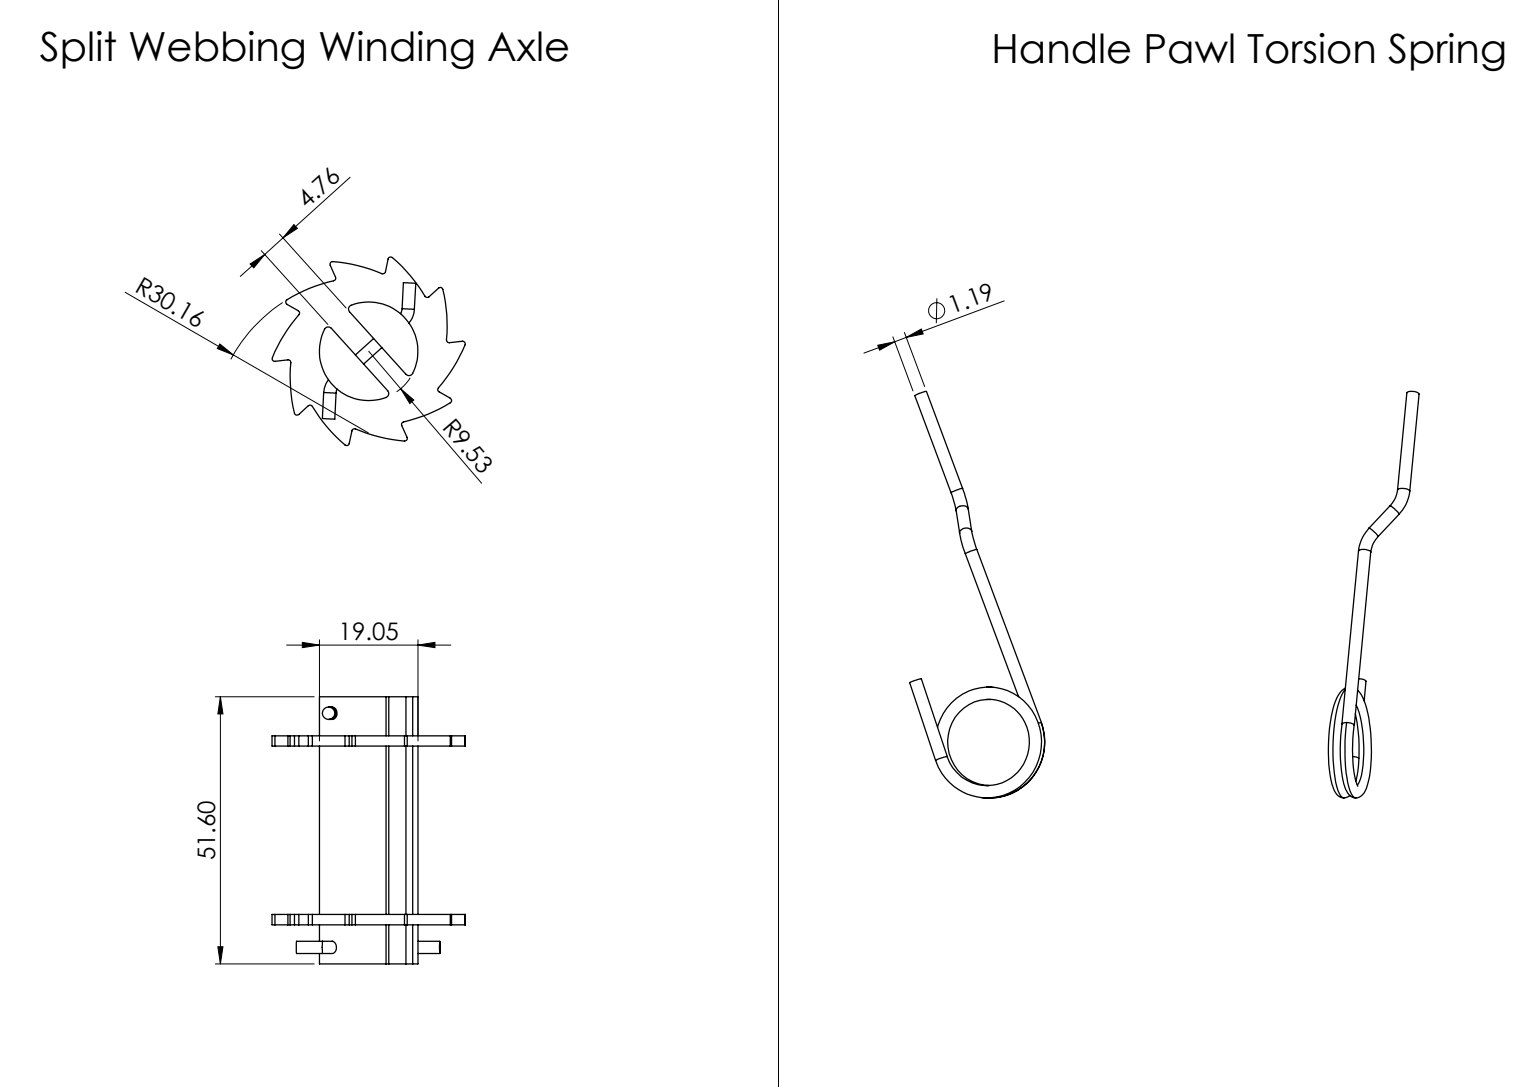
ISO-10303-21;
HEADER;
FILE_DESCRIPTION (('STEP AP214'),
    '1' );
FILE_NAME ('Split Webbing Winding Axle.step',
    '2026-10-09T14:10:49',
    ( '' ),
    ( '' ),
    'SwSTEP 2.0',
    'SolidWorks 2026',
    '' );
FILE_SCHEMA (( 'AUTOMOTIVE_DESIGN' ));
ENDSEC;

DATA;
#3=CIRCLE ( 'NONE', #8469, 0.5080000000000013394 ) ;
#24=CYLINDRICAL_SURFACE ( 'NONE', #13892, 30.16250000000000142 ) ;
#26=EDGE_CURVE ( 'NONE', #12400, #1617, #15318, .T. ) ;
#27=ORIENTED_EDGE ( 'NONE', *, *, #3397, .F. ) ;
#29=CARTESIAN_POINT ( 'NONE',  ( 53.08681243026497043, 37.69777154208443193, -16.72443647847455850 ) ) ;
#32=ORIENTED_EDGE ( 'NONE', *, *, #21036, .F. ) ;
#34=DIRECTION ( 'NONE',  ( 0.9943660382494290406, 0.000000000000000000, -0.1060008583745199739 ) ) ;
#36=EDGE_CURVE ( 'NONE', #1582, #17060, #15097, .T. ) ;
#41=ORIENTED_EDGE ( 'NONE', *, *, #3166, .F. ) ;
#52=EDGE_CURVE ( 'NONE', #9108, #5857, #17721, .T. ) ;
#53=CARTESIAN_POINT ( 'NONE',  ( 55.27198911326564001, 34.52875999999999834, 2.462719476673013830 ) ) ;
#55=ORIENTED_EDGE ( 'NONE', *, *, #21504, .F. ) ;
#56=ORIENTED_EDGE ( 'NONE', *, *, #17494, .T. ) ;
#58=CARTESIAN_POINT ( 'NONE',  ( 47.00675968526287818, 38.88803500000000213, -12.79836188810822328 ) ) ;
#62=ORIENTED_EDGE ( 'NONE', *, *, #7822, .T. ) ;
#64=VECTOR ( 'NONE', #8370, 1000.000000000000000 ) ;
#68=EDGE_CURVE ( 'NONE', #10096, #18019, #3909, .T. ) ;
#72=CYLINDRICAL_SURFACE ( 'NONE', #449, 30.16250000000000142 ) ;
#77=CYLINDRICAL_SURFACE ( 'NONE', #10849, 0.5080000000000005622 ) ;
#79=ORIENTED_EDGE ( 'NONE', *, *, #17597, .T. ) ;
#80=DIRECTION ( 'NONE',  ( 0.000000000000000000, 1.000000000000000000, 0.000000000000000000 ) ) ;
#89=ORIENTED_EDGE ( 'NONE', *, *, #190, .T. ) ;
#92=CARTESIAN_POINT ( 'NONE',  ( 39.27728671717661513, 34.52875999999999834, -23.95520057284206672 ) ) ;
#95=ORIENTED_EDGE ( 'NONE', *, *, #5447, .T. ) ;
#97=VERTEX_POINT ( 'NONE', #18926 ) ;
#101=DIRECTION ( 'NONE',  ( -0.6702301885068630005, 0.000000000000000000, -0.7421532822901580895 ) ) ;
#102=VECTOR ( 'NONE', #21181, 1000.000000000000114 ) ;
#106=FACE_OUTER_BOUND ( 'NONE', #16454, .T. ) ;
#107=VERTEX_POINT ( 'NONE', #482 ) ;
#110=CARTESIAN_POINT ( 'NONE',  ( 53.77834614425744064, -5.598900522968899729, -15.87027249378376936 ) ) ;
#112=CYLINDRICAL_SURFACE ( 'NONE', #2785, 0.5079999999999976756 ) ;
#114=EDGE_CURVE ( 'NONE', #97, #11029, #5668, .T. ) ;
#116=AXIS2_PLACEMENT_3D ( 'NONE', #2669, #1515, #18221 ) ;
#119=VERTEX_POINT ( 'NONE', #18820 ) ;
#137=EDGE_CURVE ( 'NONE', #6597, #20373, #21240, .T. ) ;
#139=DIRECTION ( 'NONE',  ( 0.05085730733808393328, 0.000000000000000000, -0.9987059298363656357 ) ) ;
#142=ORIENTED_EDGE ( 'NONE', *, *, #11602, .F. ) ;
#146=LINE ( 'NONE', #8543, #21177 ) ;
#147=VECTOR ( 'NONE', #5994, 1000.000000000000114 ) ;
#148=ORIENTED_EDGE ( 'NONE', *, *, #13327, .T. ) ;
#165=EDGE_CURVE ( 'NONE', #19859, #2625, #8173, .T. ) ;
#166=ORIENTED_EDGE ( 'NONE', *, *, #3462, .T. ) ;
#170=VECTOR ( 'NONE', #3329, 1000.000000000000000 ) ;
#173=LINE ( 'NONE', #16974, #9614 ) ;
#175=DIRECTION ( 'NONE',  ( -0.1060008583745224581, 0.000000000000000000, -0.9943660382494288186 ) ) ;
#180=VERTEX_POINT ( 'NONE', #9193 ) ;
#182=ADVANCED_FACE ( 'NONE', ( #3687 ), #8750, .T. ) ;
#185=LINE ( 'NONE', #17106, #9522 ) ;
#188=CYLINDRICAL_SURFACE ( 'NONE', #17566, 0.5080000000000007843 ) ;
#189=ORIENTED_EDGE ( 'NONE', *, *, #13845, .T. ) ;
#190=EDGE_CURVE ( 'NONE', #7494, #14487, #7555, .T. ) ;
#191=CARTESIAN_POINT ( 'NONE',  ( 53.25483508941461963, 42.06303499999999929, -5.879799058943532941 ) ) ;
#204=ORIENTED_EDGE ( 'NONE', *, *, #16141, .T. ) ;
#210=EDGE_CURVE ( 'NONE', #9895, #180, #14097, .T. ) ;
#213=DIRECTION ( 'NONE',  ( 0.2064631973582987667, 0.000000000000000000, -0.9784543669157944601 ) ) ;
#220=DIRECTION ( 'NONE',  ( 0.000000000000000000, -1.000000000000000000, 0.000000000000000000 ) ) ;
#221=CYLINDRICAL_SURFACE ( 'NONE', #1464, 0.5079999999999963434 ) ;
#225=CARTESIAN_POINT ( 'NONE',  ( 64.14292646034530776, 0.000000000000000000, -12.24881465648521939 ) ) ;
#229=CARTESIAN_POINT ( 'NONE',  ( 38.18512253410862201, -6.356984999999999886, -4.927479914652648674 ) ) ;
#248=CARTESIAN_POINT ( 'NONE',  ( 53.46798503507454825, 34.52875999999999834, 6.304111036318381878 ) ) ;
#250=FACE_OUTER_BOUND ( 'NONE', #17892, .T. ) ;
#251=ORIENTED_EDGE ( 'NONE', *, *, #17974, .F. ) ;
#253=AXIS2_PLACEMENT_3D ( 'NONE', #9461, #16230, #5826 ) ;
#261=EDGE_CURVE ( 'NONE', #11029, #831, #7657, .T. ) ;
#268=CIRCLE ( 'NONE', #3100, 1.190624999999997824 ) ;
#273=ORIENTED_EDGE ( 'NONE', *, *, #1147, .T. ) ;
#284=VECTOR ( 'NONE', #21016, 1000.000000000000000 ) ;
#286=EDGE_CURVE ( 'NONE', #20627, #1656, #19688, .T. ) ;
#293=CARTESIAN_POINT ( 'NONE',  ( 49.41195815393805901, -1.983739999999997838, -1.411525001868561224 ) ) ;
#297=ORIENTED_EDGE ( 'NONE', *, *, #14274, .F. ) ;
#299=DIRECTION ( 'NONE',  ( -0.5222415575336509797, 0.000000000000000000, -0.8527976052879290281 ) ) ;
#302=CARTESIAN_POINT ( 'NONE',  ( 32.18388890846549799, 32.54502000000000095, 1.507793899792891468 ) ) ;
#305=EDGE_LOOP ( 'NONE', ( #11333, #11552, #10599, #2404 ) ) ;
#312=ORIENTED_EDGE ( 'NONE', *, *, #165, .T. ) ;
#314=ORIENTED_EDGE ( 'NONE', *, *, #1169, .F. ) ;
#321=DIRECTION ( 'NONE',  ( 0.000000000000000000, 1.000000000000000000, 0.000000000000000000 ) ) ;
#325=CARTESIAN_POINT ( 'NONE',  ( 39.16413618835606769, 37.11476346399999926, -24.45043885672975392 ) ) ;
#330=DIRECTION ( 'NONE',  ( 0.000000000000000000, 1.000000000000000000, 0.000000000000000000 ) ) ;
#331=ORIENTED_EDGE ( 'NONE', *, *, #18672, .F. ) ;
#335=ORIENTED_EDGE ( 'NONE', *, *, #14252, .F. ) ;
#342=DIRECTION ( 'NONE',  ( -0.6496772031432439531, 0.000000000000000000, 0.7602101891687401691 ) ) ;
#343=AXIS2_PLACEMENT_3D ( 'NONE', #9406, #14736, #16073 ) ;
#346=VECTOR ( 'NONE', #19998, 1000.000000000000114 ) ;
#348=CARTESIAN_POINT ( 'NONE',  ( 38.84235393761607469, -5.162860800152350826, -4.075279525839791361 ) ) ;
#360=EDGE_CURVE ( 'NONE', #21347, #13814, #17389, .T. ) ;
#371=DIRECTION ( 'NONE',  ( -0.7421532822901579785, 0.000000000000000000, 0.6702301885068630005 ) ) ;
#373=CARTESIAN_POINT ( 'NONE',  ( 41.45112526417833010, -1.983739999999999837, 7.778260066349530710 ) ) ;
#392=DIRECTION ( 'NONE',  ( -0.7421532822901579785, 0.000000000000000000, 0.6702301885068628895 ) ) ;
#400=ORIENTED_EDGE ( 'NONE', *, *, #7902, .F. ) ;
#401=VECTOR ( 'NONE', #4265, 1000.000000000000000 ) ;
#404=ORIENTED_EDGE ( 'NONE', *, *, #18172, .T. ) ;
#405=LINE ( 'NONE', #7160, #11390 ) ;
#406=DIRECTION ( 'NONE',  ( -0.05085730733808142834, 0.000000000000000000, 0.9987059298363657467 ) ) ;
#409=CARTESIAN_POINT ( 'NONE',  ( 64.66604708500285881, 32.54502000000000095, -11.54913207920052720 ) ) ;
#412=ORIENTED_EDGE ( 'NONE', *, *, #11806, .F. ) ;
#424=LINE ( 'NONE', #13819, #15988 ) ;
#430=AXIS2_PLACEMENT_3D ( 'NONE', #13044, #6387, #21198 ) ;
#434=CIRCLE ( 'NONE', #1505, 0.5080000000000006732 ) ;
#439=DIRECTION ( 'NONE',  ( 0.8943161143440100380, 0.000000000000000000, 0.4474356798743612806 ) ) ;
#449=AXIS2_PLACEMENT_3D ( 'NONE', #12581, #16021, #15571 ) ;
#450=ORIENTED_EDGE ( 'NONE', *, *, #19358, .T. ) ;
#454=EDGE_CURVE ( 'NONE', #9720, #5388, #7845, .T. ) ;
#455=DIRECTION ( 'NONE',  ( 0.000000000000000000, 1.000000000000000000, 0.000000000000000000 ) ) ;
#459=CIRCLE ( 'NONE', #9260, 0.5079999999999973426 ) ;
#477=PLANE ( 'NONE',  #19448 ) ;
#482=CARTESIAN_POINT ( 'NONE',  ( 30.97944403357121956, -1.983739999999999837, -8.103300075789407586 ) ) ;
#485=ORIENTED_EDGE ( 'NONE', *, *, #3071, .F. ) ;
#493=CIRCLE ( 'NONE', #844, 1.190625000000000711 ) ;
#498=EDGE_CURVE ( 'NONE', #10812, #21347, #20182, .T. ) ;
#499=CARTESIAN_POINT ( 'NONE',  ( 53.14266576735298031, -7.546379553159687781, -16.66242751532464084 ) ) ;
#504=CARTESIAN_POINT ( 'NONE',  ( 52.39214030333819494, 39.62760010306434566, -17.41425762687993029 ) ) ;
#512=DIRECTION ( 'NONE',  ( 0.1060008583745224581, 0.000000000000000000, 0.9943660382494288186 ) ) ;
#521=AXIS2_PLACEMENT_3D ( 'NONE', #15161, #6738, #13502 ) ;
#523=DIRECTION ( 'NONE',  ( 0.7421532822901579785, 0.000000000000000000, -0.6702301885068630005 ) ) ;
#524=EDGE_LOOP ( 'NONE', ( #10286, #14452, #3255, #19034 ) ) ;
#525=CARTESIAN_POINT ( 'NONE',  ( 59.65121809612895731, 0.000000000000000000, -2.485718937265306572 ) ) ;
#527=CARTESIAN_POINT ( 'NONE',  ( 59.86950051480232560, -6.356984999999999886, -17.89453710146031185 ) ) ;
#530=ORIENTED_EDGE ( 'NONE', *, *, #8325, .F. ) ;
#531=ORIENTED_EDGE ( 'NONE', *, *, #4323, .T. ) ;
#535=VERTEX_POINT ( 'NONE', #17898 ) ;
#538=ORIENTED_EDGE ( 'NONE', *, *, #3166, .T. ) ;
#541=AXIS2_PLACEMENT_3D ( 'NONE', #1411, #17800, #2648 ) ;
#542=ORIENTED_EDGE ( 'NONE', *, *, #52, .F. ) ;
#546=CARTESIAN_POINT ( 'NONE',  ( 38.94885947252247860, -7.547248457916676756, -3.956611957470116625 ) ) ;
#551=DIRECTION ( 'NONE',  ( 0.000000000000000000, -1.000000000000000000, 0.000000000000000000 ) ) ;
#553=DIRECTION ( 'NONE',  ( -0.8583349619704310207, 0.000000000000000000, 0.5130897514657826175 ) ) ;
#557=ORIENTED_EDGE ( 'NONE', *, *, #19024, .T. ) ;
#563=ORIENTED_EDGE ( 'NONE', *, *, #17228, .T. ) ;
#568=CARTESIAN_POINT ( 'NONE',  ( 64.14292646034530776, -1.983739999999999837, -12.24881465648521939 ) ) ;
#570=EDGE_CURVE ( 'NONE', #16730, #6476, #8894, .T. ) ;
#575=ADVANCED_FACE ( 'NONE', ( #16250 ), #19549, .F. ) ;
#584=CARTESIAN_POINT ( 'NONE',  ( 52.91086381164393515, 2.586003464000000029, 3.812938856729753301 ) ) ;
#589=LINE ( 'NONE', #20695, #6002 ) ;
#597=EDGE_CURVE ( 'NONE', #14787, #535, #13511, .T. ) ;
#602=DIRECTION ( 'NONE',  ( 0.9129422336036122632, 0.000000000000000000, -0.4080888115384288528 ) ) ;
#609=ORIENTED_EDGE ( 'NONE', *, *, #4647, .F. ) ;
#611=CARTESIAN_POINT ( 'NONE',  ( 30.25543876212147509, 34.52875999999999834, -19.39939755251907272 ) ) ;
#614=FACE_OUTER_BOUND ( 'NONE', #18678, .T. ) ;
#619=CYLINDRICAL_SURFACE ( 'NONE', #19701, 30.16249999999999076 ) ;
#620=EDGE_CURVE ( 'NONE', #8192, #8377, #16467, .T. ) ;
#621=EDGE_LOOP ( 'NONE', ( #5754, #17722, #15374, #17996, #9493, #4829, #6803, #12935, #19285, #5126, #563, #5731, #12820, #9699, #14120, #19790, #20475, #19543, #9154, #13893, #19426, #8672, #3701, #4027, #204, #17065, #19652, #9741, #16692, #2515, #19472, #8946, #13944, #4403, #14015, #10589, #1724, #609, #18551, #13398 ) ) ;
#625=CARTESIAN_POINT ( 'NONE',  ( 59.80894853325292360, -6.356984999999999886, -16.70545285374888778 ) ) ;
#633=AXIS2_PLACEMENT_3D ( 'NONE', #13523, #13632, #8307 ) ;
#651=ORIENTED_EDGE ( 'NONE', *, *, #18149, .F. ) ;
#661=DIRECTION ( 'NONE',  ( 0.07875956036501312318, 0.000000000000000000, -0.9968936410927243807 ) ) ;
#667=CIRCLE ( 'NONE', #3491, 1.984375000000000000 ) ;
#672=CARTESIAN_POINT ( 'NONE',  ( 37.13209340688868565, -6.356984999999999886, -3.529402718062123689 ) ) ;
#673=VECTOR ( 'NONE', #3578, 1000.000000000000000 ) ;
#683=DIRECTION ( 'NONE',  ( 0.000000000000000000, 1.000000000000000000, 0.000000000000000000 ) ) ;
#684=CARTESIAN_POINT ( 'NONE',  ( 38.23013820809905638, -9.531985000000000596, -14.22485453658974031 ) ) ;
#687=AXIS2_PLACEMENT_3D ( 'NONE', #15125, #6696, #20168 ) ;
#689=ORIENTED_EDGE ( 'NONE', *, *, #13845, .F. ) ;
#690=DIRECTION ( 'NONE',  ( -0.000000000000000000, -1.000000000000000000, 0.000000000000000000 ) ) ;
#704=DIRECTION ( 'NONE',  ( 0.9784543669157820256, 0.000000000000000000, 0.2064631973583577473 ) ) ;
#709=VECTOR ( 'NONE', #2797, 1000.000000000000000 ) ;
#713=FACE_OUTER_BOUND ( 'NONE', #15999, .T. ) ;
#715=ADVANCED_FACE ( 'NONE', ( #13584 ), #1729, .F. ) ;
#718=ADVANCED_FACE ( 'NONE', ( #1946 ), #18430, .T. ) ;
#719=ADVANCED_FACE ( 'NONE', ( #3305 ), #10243, .F. ) ;
#723=VERTEX_POINT ( 'NONE', #3504 ) ;
#734=DIRECTION ( 'NONE',  ( 0.3928209820863007851, 0.000000000000000000, -0.9196149607486571176 ) ) ;
#741=ORIENTED_EDGE ( 'NONE', *, *, #1772, .T. ) ;
#745=LINE ( 'NONE', #16241, #21205 ) ;
#746=CIRCLE ( 'NONE', #9211, 0.5079999999999996740 ) ;
#747=EDGE_LOOP ( 'NONE', ( #450, #19069, #6393, #18964 ) ) ;
#753=ORIENTED_EDGE ( 'NONE', *, *, #1834, .F. ) ;
#756=CIRCLE ( 'NONE', #19475, 0.5079999999999985638 ) ;
#758=EDGE_CURVE ( 'NONE', #20373, #1329, #18433, .T. ) ;
#763=AXIS2_PLACEMENT_3D ( 'NONE', #1873, #5290, #4872 ) ;
#770=CARTESIAN_POINT ( 'NONE',  ( 55.33978576324753362, 0.000000000000000000, -23.05096232720518756 ) ) ;
#774=DIRECTION ( 'NONE',  ( 0.000000000000000000, 1.000000000000000000, 0.000000000000000000 ) ) ;
#780=DIRECTION ( 'NONE',  ( 0.000000000000000000, 1.000000000000000000, 0.000000000000000000 ) ) ;
#781=AXIS2_PLACEMENT_3D ( 'NONE', #4089, #977, #12506 ) ;
#782=AXIS2_PLACEMENT_3D ( 'NONE', #19094, #1965, #3522 ) ;
#784=DIRECTION ( 'NONE',  ( 0.000000000000000000, 1.000000000000000000, 0.000000000000000000 ) ) ;
#789=AXIS2_PLACEMENT_3D ( 'NONE', #10505, #19118, #10616 ) ;
#790=CARTESIAN_POINT ( 'NONE',  ( 38.23013820809905638, 42.06303499999999929, -14.22485453658974031 ) ) ;
#791=DIRECTION ( 'NONE',  ( -0.4080888115384288528, 0.000000000000000000, -0.9129422336036122632 ) ) ;
#804=DIRECTION ( 'NONE',  ( 0.000000000000000000, 1.000000000000000000, 0.000000000000000000 ) ) ;
#806=VECTOR ( 'NONE', #16119, 1000.000000000000000 ) ;
#809=DIRECTION ( 'NONE',  ( 0.000000000000000000, 1.000000000000000000, 0.000000000000000000 ) ) ;
#819=ORIENTED_EDGE ( 'NONE', *, *, #16382, .T. ) ;
#824=DIRECTION ( 'NONE',  ( -0.1060008583745224581, 0.000000000000000000, -0.9943660382494288186 ) ) ;
#826=PRODUCT_DEFINITION_CONTEXT ( 'detailed design', #18349, 'design' ) ;
#830=CARTESIAN_POINT ( 'NONE',  ( 52.22368883687065022, 39.20681492737163154, -17.56171959381228476 ) ) ;
#831=VERTEX_POINT ( 'NONE', #12016 ) ;
#834=CIRCLE ( 'NONE', #8244, 30.16249999999998721 ) ;
#837=CARTESIAN_POINT ( 'NONE',  ( 59.52193197173441774, -1.983739999999999837, -3.260183413611184911 ) ) ;
#838=ORIENTED_EDGE ( 'NONE', *, *, #9399, .T. ) ;
#841=ORIENTED_EDGE ( 'NONE', *, *, #10075, .F. ) ;
#844=AXIS2_PLACEMENT_3D ( 'NONE', #8969, #14195, #20909 ) ;
#850=ADVANCED_FACE ( 'NONE', ( #10135 ), #72, .T. ) ;
#855=LINE ( 'NONE', #17779, #102 ) ;
#856=CARTESIAN_POINT ( 'NONE',  ( 38.94885947252247860, -7.547248457916676756, -3.956611957470116625 ) ) ;
#858=ORIENTED_EDGE ( 'NONE', *, *, #4636, .F. ) ;
#859=ORIENTED_EDGE ( 'NONE', *, *, #3535, .T. ) ;
#863=ORIENTED_EDGE ( 'NONE', *, *, #16462, .T. ) ;
#866=ORIENTED_EDGE ( 'NONE', *, *, #19505, .T. ) ;
#867=VECTOR ( 'NONE', #15872, 1000.000000000000000 ) ;
#872=EDGE_CURVE ( 'NONE', #8553, #5503, #6086, .T. ) ;
#874=CARTESIAN_POINT ( 'NONE',  ( 59.55063415577301811, 32.54502000000000095, -22.52230776719629191 ) ) ;
#877=VERTEX_POINT ( 'NONE', #9239 ) ;
#881=CYLINDRICAL_SURFACE ( 'NONE', #9261, 1.190624999999997824 ) ;
#890=VECTOR ( 'NONE', #9483, 1000.000000000000000 ) ;
#895=CARTESIAN_POINT ( 'NONE',  ( 59.90456643211351917, 37.11476346399999926, -2.926035437812116946 ) ) ;
#900=DIRECTION ( 'NONE',  ( 0.000000000000000000, 1.000000000000000000, 0.000000000000000000 ) ) ;
#906=FACE_OUTER_BOUND ( 'NONE', #1227, .T. ) ;
#909=DIRECTION ( 'NONE',  ( 0.000000000000000000, -1.000000000000000000, -0.000000000000000000 ) ) ;
#914=EDGE_LOOP ( 'NONE', ( #6101, #19962 ) ) ;
#917=LINE ( 'NONE', #20928, #8769 ) ;
#923=CARTESIAN_POINT ( 'NONE',  ( 53.00421038040393995, 0.000000000000000000, 6.511420152579801446 ) ) ;
#924=ORIENTED_EDGE ( 'NONE', *, *, #3296, .T. ) ;
#929=CARTESIAN_POINT ( 'NONE',  ( 53.50176854207381183, -7.446663216667899654, -16.23620094008295567 ) ) ;
#930=CARTESIAN_POINT ( 'NONE',  ( 39.90410341501912939, 39.21273375806297423, -3.030981210009983329 ) ) ;
#933=ORIENTED_EDGE ( 'NONE', *, *, #3535, .F. ) ;
#934=CARTESIAN_POINT ( 'NONE',  ( 52.55824432597118800, 39.85392714130129832, -17.26273071540813930 ) ) ;
#935=ORIENTED_EDGE ( 'NONE', *, *, #8739, .T. ) ;
#940=CARTESIAN_POINT ( 'NONE',  ( 38.23013820809905638, 109.3223030719999969, -14.22485453658974031 ) ) ;
#948=ORIENTED_EDGE ( 'NONE', *, *, #19907, .F. ) ;
#953=CYLINDRICAL_SURFACE ( 'NONE', #8579, 1.190624999999999822 ) ;
#954=DIRECTION ( 'NONE',  ( 0.000000000000000000, 1.000000000000000000, 0.000000000000000000 ) ) ;
#964=EDGE_CURVE ( 'NONE', #12607, #1384, #20908, .T. ) ;
#965=CIRCLE ( 'NONE', #18263, 4.365624999999999645 ) ;
#968=VERTEX_POINT ( 'NONE', #12242 ) ;
#970=FACE_OUTER_BOUND ( 'NONE', #7558, .T. ) ;
#976=DIRECTION ( 'NONE',  ( -0.9987059298363656357, 0.000000000000000000, -0.05085730733808393328 ) ) ;
#977=DIRECTION ( 'NONE',  ( 0.000000000000000000, 1.000000000000000000, 0.000000000000000000 ) ) ;
#981=ORIENTED_EDGE ( 'NONE', *, *, #3143, .F. ) ;
#991=DIRECTION ( 'NONE',  ( 0.000000000000000000, 1.000000000000000000, 0.000000000000000000 ) ) ;
#994=VECTOR ( 'NONE', #12853, 1000.000000000000000 ) ;
#1006=LINE ( 'NONE', #14849, #1063 ) ;
#1009=EDGE_CURVE ( 'NONE', #968, #19531, #14254, .T. ) ;
#1011=CARTESIAN_POINT ( 'NONE',  ( 61.65536943582333151, 0.000000000000000000, -11.98363747855214712 ) ) ;
#1021=VERTEX_POINT ( 'NONE', #8792 ) ;
#1028=DIRECTION ( 'NONE',  ( 0.000000000000000000, -1.000000000000000000, -0.000000000000000000 ) ) ;
#1030=DIRECTION ( 'NONE',  ( 0.000000000000000000, -1.000000000000000000, -0.000000000000000000 ) ) ;
#1033=EDGE_CURVE ( 'NONE', #1535, #12957, #405, .T. ) ;
#1034=VECTOR ( 'NONE', #2801, 1000.000000000000114 ) ;
#1038=DIRECTION ( 'NONE',  ( 0.000000000000000000, -1.000000000000000000, -0.000000000000000000 ) ) ;
#1039=DIRECTION ( 'NONE',  ( 0.000000000000000000, 1.000000000000000000, 0.000000000000000000 ) ) ;
#1042=CARTESIAN_POINT ( 'NONE',  ( 53.10651001381376091, 37.69740999999999786, -16.70269254552787075 ) ) ;
#1046=LINE ( 'NONE', #9338, #10598 ) ;
#1050=VERTEX_POINT ( 'NONE', #12996 ) ;
#1060=EDGE_CURVE ( 'NONE', #11223, #2583, #1466, .T. ) ;
#1063=VECTOR ( 'NONE', #5977, 1000.000000000000114 ) ;
#1065=VECTOR ( 'NONE', #13779, 1000.000000000000000 ) ;
#1068=VERTEX_POINT ( 'NONE', #18065 ) ;
#1074=VERTEX_POINT ( 'NONE', #6656 ) ;
#1075=AXIS2_PLACEMENT_3D ( 'NONE', #5417, #7209, #5200 ) ;
#1078=AXIS2_PLACEMENT_3D ( 'NONE', #1933, #7356, #5576 ) ;
#1081=CARTESIAN_POINT ( 'NONE',  ( 39.54651519818619221, 37.91656218874415885, -3.347550931093328686 ) ) ;
#1089=TOROIDAL_SURFACE ( 'NONE', #15240, 3.174999999999999822, 1.190625000000000044 ) ;
#1095=ORIENTED_EDGE ( 'NONE', *, *, #21176, .F. ) ;
#1099=CARTESIAN_POINT ( 'NONE',  ( 36.80301088673436283, 0.000000000000000000, -23.10021947667301134 ) ) ;
#1112=DIRECTION ( 'NONE',  ( -0.9129422336036127072, 0.000000000000000000, 0.4080888115384278536 ) ) ;
#1116=EDGE_CURVE ( 'NONE', #20800, #15003, #18486, .T. ) ;
#1117=VERTEX_POINT ( 'NONE', #11433 ) ;
#1123=DIRECTION ( 'NONE',  ( -0.3928209820863007296, 0.000000000000000000, 0.9196149607486571176 ) ) ;
#1124=AXIS2_PLACEMENT_3D ( 'NONE', #1554, #6631, #4975 ) ;
#1126=VERTEX_POINT ( 'NONE', #8214 ) ;
#1128=AXIS2_PLACEMENT_3D ( 'NONE', #3087, #5065, #9811 ) ;
#1136=CARTESIAN_POINT ( 'NONE',  ( 39.88301061098722755, 0.000000000000000000, -24.08706006053352411 ) ) ;
#1137=EDGE_CURVE ( 'NONE', #8133, #7171, #5738, .T. ) ;
#1144=CARTESIAN_POINT ( 'NONE',  ( 45.99559936598748777, 34.52875999999999834, 5.449572532947073000 ) ) ;
#1146=AXIS2_PLACEMENT_3D ( 'NONE', #16018, #14139, #3837 ) ;
#1147=EDGE_CURVE ( 'NONE', #1819, #7588, #4799, .T. ) ;
#1163=CARTESIAN_POINT ( 'NONE',  ( 49.79678389823170903, 34.52875999999999834, -28.13445659451038594 ) ) ;
#1166=ADVANCED_FACE ( 'NONE', ( #13103 ), #1350, .T. ) ;
#1169=EDGE_CURVE ( 'NONE', #1190, #8553, #3129, .T. ) ;
#1174=AXIS2_PLACEMENT_3D ( 'NONE', #20913, #5776, #4011 ) ;
#1175=CARTESIAN_POINT ( 'NONE',  ( 38.76261520251843251, 37.72836252664282597, -4.168749548257426163 ) ) ;
#1181=CARTESIAN_POINT ( 'NONE',  ( 38.82016491058538321, 42.06303499999999929, -14.75770094105646812 ) ) ;
#1183=ORIENTED_EDGE ( 'NONE', *, *, #18457, .T. ) ;
#1184=DIRECTION ( 'NONE',  ( 0.000000000000000000, -1.000000000000000000, -0.000000000000000000 ) ) ;
#1190=VERTEX_POINT ( 'NONE', #3244 ) ;
#1193=ADVANCED_FACE ( 'NONE', ( #6330 ), #3031, .F. ) ;
#1197=CIRCLE ( 'NONE', #13575, 0.7950199999999993938 ) ;
#1198=CARTESIAN_POINT ( 'NONE',  ( 38.18512253410862201, -6.356984999999999886, -4.927479914652648674 ) ) ;
#1199=CYLINDRICAL_SURFACE ( 'NONE', #4030, 1.190625000000000488 ) ;
#1206=DIRECTION ( 'NONE',  ( -0.3542738219355860418, 0.000000000000000000, -0.9351417320872557060 ) ) ;
#1207=CARTESIAN_POINT ( 'NONE',  ( 53.84912356528904809, 38.73144433068016923, -15.76890250127162219 ) ) ;
#1209=VERTEX_POINT ( 'NONE', #4689 ) ;
#1217=CARTESIAN_POINT ( 'NONE',  ( 32.96560389001691505, 0.000000000000000000, -17.84002872454335886 ) ) ;
#1223=CARTESIAN_POINT ( 'NONE',  ( 61.65536943582333151, -1.983739999999999837, -11.98363747855214712 ) ) ;
#1226=DIRECTION ( 'NONE',  ( -0.4987171968201974948, 0.000000000000000000, 0.8667647648559581031 ) ) ;
#1227=EDGE_LOOP ( 'NONE', ( #9061, #2863, #19485, #6400 ) ) ;
#1229=DIRECTION ( 'NONE',  ( 0.000000000000000000, 1.000000000000000000, 0.000000000000000000 ) ) ;
#1232=CIRCLE ( 'NONE', #9341, 30.16249999999999076 ) ;
#1233=CARTESIAN_POINT ( 'NONE',  ( 36.80301088673436283, 32.54502000000000095, -23.10021947667301134 ) ) ;
#1234=ORIENTED_EDGE ( 'NONE', *, *, #7163, .T. ) ;
#1235=DIRECTION ( 'NONE',  ( -0.2227372614607789347, 0.000000000000000000, -0.9748785115884710528 ) ) ;
#1241=DIRECTION ( 'NONE',  ( 0.4987171968201974948, 0.000000000000000000, -0.8667647648559581031 ) ) ;
#1244=EDGE_CURVE ( 'NONE', #3969, #9951, #4333, .T. ) ;
#1245=ADVANCED_FACE ( 'NONE', ( #4575 ), #11315, .T. ) ;
#1247=DIRECTION ( 'NONE',  ( 0.7532174416907910786, 0.000000000000000000, 0.6577716059034319773 ) ) ;
#1251=CARTESIAN_POINT ( 'NONE',  ( 35.15748561355322011, -1.983739999999999837, 0.3244898641346534163 ) ) ;
#1254=CARTESIAN_POINT ( 'NONE',  ( 39.22869158989735894, 40.05999463121278836, -3.656238088543281695 ) ) ;
#1258=EDGE_CURVE ( 'NONE', #8259, #8918, #16003, .T. ) ;
#1263=DIRECTION ( 'NONE',  ( -0.6702301885068630005, 0.000000000000000000, -0.7421532822901579785 ) ) ;
#1265=PLANE ( 'NONE',  #7770 ) ;
#1271=EDGE_CURVE ( 'NONE', #1509, #15569, #7226, .T. ) ;
#1277=ADVANCED_FACE ( 'NONE', ( #20683 ), #18810, .T. ) ;
#1278=CARTESIAN_POINT ( 'NONE',  ( 38.22590828043067290, 38.73299043104906758, -4.868551855887884194 ) ) ;
#1283=ORIENTED_EDGE ( 'NONE', *, *, #9674, .T. ) ;
#1284=FACE_OUTER_BOUND ( 'NONE', #12717, .T. ) ;
#1287=ORIENTED_EDGE ( 'NONE', *, *, #8664, .T. ) ;
#1288=EDGE_CURVE ( 'NONE', #2524, #17693, #18696, .T. ) ;
#1289=ORIENTED_EDGE ( 'NONE', *, *, #16141, .F. ) ;
#1293=ORIENTED_EDGE ( 'NONE', *, *, #4679, .T. ) ;
#1296=ORIENTED_EDGE ( 'NONE', *, *, #11249, .T. ) ;
#1301=PLANE ( 'NONE',  #11805 ) ;
#1304=ORIENTED_EDGE ( 'NONE', *, *, #18290, .T. ) ;
#1306=CARTESIAN_POINT ( 'NONE',  ( 46.03750000000000142, 0.000000000000000000, -10.31874999999999964 ) ) ;
#1312=ORIENTED_EDGE ( 'NONE', *, *, #21259, .T. ) ;
#1315=CARTESIAN_POINT ( 'NONE',  ( 64.19677489640052670, 32.54502000000000095, -11.74367670905533423 ) ) ;
#1323=AXIS2_PLACEMENT_3D ( 'NONE', #10611, #20419, #3763 ) ;
#1325=DIRECTION ( 'NONE',  ( 0.000000000000000000, -1.000000000000000000, -0.000000000000000000 ) ) ;
#1329=VERTEX_POINT ( 'NONE', #6092 ) ;
#1332=FACE_OUTER_BOUND ( 'NONE', #2278, .T. ) ;
#1340=AXIS2_PLACEMENT_3D ( 'NONE', #2556, #12406, #17593 ) ;
#1342=CARTESIAN_POINT ( 'NONE',  ( 53.25483508941461963, -9.531985000000000596, -5.879799058943532941 ) ) ;
#1350=CYLINDRICAL_SURFACE ( 'NONE', #3619, 0.5079999999999965654 ) ;
#1353=LINE ( 'NONE', #21593, #9596 ) ;
#1357=CARTESIAN_POINT ( 'NONE',  ( 61.60152099976809126, -1.983739999999999837, -12.48877542598203405 ) ) ;
#1358=CARTESIAN_POINT ( 'NONE',  ( 64.66604708500285881, -1.983739999999999837, -11.54913207920052720 ) ) ;
#1362=CARTESIAN_POINT ( 'NONE',  ( 61.56621290189396944, 34.52875999999999834, -0.7977859469341201937 ) ) ;
#1363=CARTESIAN_POINT ( 'NONE',  ( 52.55890053324426248, 37.92160077886185121, -17.26210851293683390 ) ) ;
#1370=CARTESIAN_POINT ( 'NONE',  ( 42.79471501377724252, 34.52875999999999834, 5.049205022181460834 ) ) ;
#1382=( NAMED_UNIT ( * ) PLANE_ANGLE_UNIT ( ) SI_UNIT ( $, .RADIAN. ) );
#1383=ADVANCED_FACE ( 'NONE', ( #906 ), #2456, .F. ) ;
#1384=VERTEX_POINT ( 'NONE', #2567 ) ;
#1398=ORIENTED_EDGE ( 'NONE', *, *, #18691, .F. ) ;
#1400=CIRCLE ( 'NONE', #10270, 0.5080000000000016724 ) ;
#1411=CARTESIAN_POINT ( 'NONE',  ( 46.07940063401251507, 0.000000000000000000, -26.08707253294707229 ) ) ;
#1415=EDGE_CURVE ( 'NONE', #7335, #3338, #5734, .T. ) ;
#1416=LINE ( 'NONE', #8050, #20933 ) ;
#1419=CARTESIAN_POINT ( 'NONE',  ( 53.57639120092643736, 39.84016936695267930, -16.14136963297940497 ) ) ;
#1425=VERTEX_POINT ( 'NONE', #19582 ) ;
#1430=EDGE_CURVE ( 'NONE', #12951, #877, #19467, .T. ) ;
#1435=DIRECTION ( 'NONE',  ( -0.7421532822901579785, 0.000000000000000000, 0.6702301885068630005 ) ) ;
#1456=DIRECTION ( 'NONE',  ( 0.7421532822901579785, 0.000000000000000000, -0.6702301885068630005 ) ) ;
#1459=AXIS2_PLACEMENT_3D ( 'NONE', #6311, #9520, #1123 ) ;
#1463=CARTESIAN_POINT ( 'NONE',  ( 52.79771328282338771, 0.000000000000000000, 3.317700572842066986 ) ) ;
#1464=AXIS2_PLACEMENT_3D ( 'NONE', #18570, #6861, #6961 ) ;
#1465=AXIS2_PLACEMENT_3D ( 'NONE', #8510, #8080, #8195 ) ;
#1466=LINE ( 'NONE', #6450, #2210 ) ;
#1467=LINE ( 'NONE', #7779, #17824 ) ;
#1470=CARTESIAN_POINT ( 'NONE',  ( 54.55586098912687731, 42.06303499999999929, -6.056925149195119040 ) ) ;
#1471=AXIS2_PLACEMENT_3D ( 'NONE', #4974, #20002, #14962 ) ;
#1475=LINE ( 'NONE', #8221, #9766 ) ;
#1482=CYLINDRICAL_SURFACE ( 'NONE', #18394, 0.7950199999999985057 ) ;
#1485=ORIENTED_EDGE ( 'NONE', *, *, #2953, .T. ) ;
#1488=CIRCLE ( 'NONE', #9595, 30.16249999999999076 ) ;
#1505=AXIS2_PLACEMENT_3D ( 'NONE', #9439, #21375, #6231 ) ;
#1508=CARTESIAN_POINT ( 'NONE',  ( 52.65345379380355695, 37.69740999999999786, -16.29354262597941982 ) ) ;
#1509=VERTEX_POINT ( 'NONE', #21425 ) ;
#1511=ORIENTED_EDGE ( 'NONE', *, *, #4111, .T. ) ;
#1512=VERTEX_POINT ( 'NONE', #13051 ) ;
#1513=AXIS2_PLACEMENT_3D ( 'NONE', #12024, #14937, #10368 ) ;
#1514=EDGE_CURVE ( 'NONE', #18977, #107, #1416, .T. ) ;
#1515=DIRECTION ( 'NONE',  ( 0.000000000000000000, 1.000000000000000000, 0.000000000000000000 ) ) ;
#1516=EDGE_LOOP ( 'NONE', ( #5996, #3693 ) ) ;
#1527=DIRECTION ( 'NONE',  ( 0.8667647648559581031, 0.000000000000000000, 0.4987171968201974948 ) ) ;
#1529=CARTESIAN_POINT ( 'NONE',  ( 53.57721252000833800, 37.93694508125481235, -16.14030231556136741 ) ) ;
#1531=ORIENTED_EDGE ( 'NONE', *, *, #360, .T. ) ;
#1535=VERTEX_POINT ( 'NONE', #11049 ) ;
#1536=ADVANCED_FACE ( 'NONE', ( #12712 ), #21206, .F. ) ;
#1538=ORIENTED_EDGE ( 'NONE', *, *, #8761, .F. ) ;
#1544=AXIS2_PLACEMENT_3D ( 'NONE', #5510, #321, #15717 ) ;
#1546=DIRECTION ( 'NONE',  ( -0.6702301885068638887, 0.000000000000000000, -0.7421532822901570903 ) ) ;
#1549=DIRECTION ( 'NONE',  ( 0.9129422336036127072, 0.000000000000000000, -0.4080888115384278536 ) ) ;
#1554=CARTESIAN_POINT ( 'NONE',  ( 47.80475250345301674, -6.356984999999999886, -11.91473563638243327 ) ) ;
#1556=ORIENTED_EDGE ( 'NONE', *, *, #5973, .T. ) ;
#1562=AXIS2_PLACEMENT_3D ( 'NONE', #2373, #4142, #10880 ) ;
#1566=FACE_OUTER_BOUND ( 'NONE', #20603, .T. ) ;
#1567=CARTESIAN_POINT ( 'NONE',  ( 41.78116128337411794, 34.52875999999999834, 7.392073290253172502 ) ) ;
#1571=ORIENTED_EDGE ( 'NONE', *, *, #1634, .T. ) ;
#1574=AXIS2_PLACEMENT_3D ( 'NONE', #19977, #2980, #16575 ) ;
#1577=CARTESIAN_POINT ( 'NONE',  ( 41.71184157647478230, 38.88803500000000213, -2.134205101306931862 ) ) ;
#1582=VERTEX_POINT ( 'NONE', #19437 ) ;
#1598=ORIENTED_EDGE ( 'NONE', *, *, #13900, .F. ) ;
#1603=AXIS2_PLACEMENT_3D ( 'NONE', #8646, #3680, #10425 ) ;
#1605=CYLINDRICAL_SURFACE ( 'NONE', #14505, 30.16250000000000497 ) ;
#1606=ORIENTED_EDGE ( 'NONE', *, *, #68, .T. ) ;
#1610=CARTESIAN_POINT ( 'NONE',  ( 53.95242430215955665, 38.88803500000000213, -23.51676380836238067 ) ) ;
#1611=ORIENTED_EDGE ( 'NONE', *, *, #18172, .F. ) ;
#1613=ADVANCED_FACE ( 'NONE', ( #17904 ), #3086, .F. ) ;
#1617=VERTEX_POINT ( 'NONE', #7833 ) ;
#1620=ORIENTED_EDGE ( 'NONE', *, *, #12085, .F. ) ;
#1621=CARTESIAN_POINT ( 'NONE',  ( 38.23013820809905638, 34.52875999999999834, -14.22485453658974031 ) ) ;
#1623=CARTESIAN_POINT ( 'NONE',  ( 49.72033008250774344, 42.06303499999999929, -2.687827786179598277 ) ) ;
#1627=DIRECTION ( 'NONE',  ( 0.5222415575336524229, 0.000000000000000000, 0.8527976052879281399 ) ) ;
#1634=EDGE_CURVE ( 'NONE', #1329, #15472, #9617, .T. ) ;
#1636=DIRECTION ( 'NONE',  ( 0.000000000000000000, 1.000000000000000000, 0.000000000000000000 ) ) ;
#1640=AXIS2_PLACEMENT_3D ( 'NONE', #18596, #3466, #10200 ) ;
#1650=EDGE_LOOP ( 'NONE', ( #3417, #10618, #16697, #7905 ) ) ;
#1653=CARTESIAN_POINT ( 'NONE',  ( 52.89438837027574181, -7.516544198863053694, -16.93158128026265885 ) ) ;
#1656=VERTEX_POINT ( 'NONE', #191 ) ;
#1670=EDGE_CURVE ( 'NONE', #1656, #13806, #15669, .T. ) ;
#1675=DIRECTION ( 'NONE',  ( 0.000000000000000000, 1.000000000000000000, 0.000000000000000000 ) ) ;
#1679=VECTOR ( 'NONE', #5420, 1000.000000000000000 ) ;
#1680=ORIENTED_EDGE ( 'NONE', *, *, #21692, .T. ) ;
#1681=EDGE_CURVE ( 'NONE', #14418, #11144, #11913, .T. ) ;
#1690=ORIENTED_EDGE ( 'NONE', *, *, #5153, .F. ) ;
#1698=VERTEX_POINT ( 'NONE', #16886 ) ;
#1701=EDGE_CURVE ( 'NONE', #13851, #8918, #7179, .T. ) ;
#1716=AXIS2_PLACEMENT_3D ( 'NONE', #4854, #11488, #15146 ) ;
#1724=ORIENTED_EDGE ( 'NONE', *, *, #15650, .T. ) ;
#1725=DIRECTION ( 'NONE',  ( 0.9959941601142464629, 0.000000000000000000, 0.08941830359784661009 ) ) ;
#1726=ORIENTED_EDGE ( 'NONE', *, *, #19630, .T. ) ;
#1727=EDGE_CURVE ( 'NONE', #6920, #17175, #14614, .T. ) ;
#1729=CYLINDRICAL_SURFACE ( 'NONE', #21257, 0.5080000000000014504 ) ;
#1732=FACE_OUTER_BOUND ( 'NONE', #14774, .T. ) ;
#1735=VERTEX_POINT ( 'NONE', #20293 ) ;
#1742=ORIENTED_EDGE ( 'NONE', *, *, #19248, .F. ) ;
#1746=ORIENTED_EDGE ( 'NONE', *, *, #14225, .F. ) ;
#1760=DIRECTION ( 'NONE',  ( 0.9784543669157820256, 0.000000000000000000, 0.2064631973583577473 ) ) ;
#1764=VECTOR ( 'NONE', #9628, 1000.000000000000000 ) ;
#1767=CIRCLE ( 'NONE', #6716, 0.5080000000000000071 ) ;
#1772=EDGE_CURVE ( 'NONE', #4527, #1656, #18757, .T. ) ;
#1773=CARTESIAN_POINT ( 'NONE',  ( 39.58386072796550081, 38.88803500000000213, -4.490541772578183100 ) ) ;
#1777=EDGE_CURVE ( 'NONE', #13169, #13930, #7878, .T. ) ;
#1787=FACE_OUTER_BOUND ( 'NONE', #13799, .T. ) ;
#1790=VECTOR ( 'NONE', #4709, 1000.000000000000000 ) ;
#1795=LINE ( 'NONE', #17058, #10488 ) ;
#1803=EDGE_CURVE ( 'NONE', #16972, #11670, #19980, .T. ) ;
#1806=VECTOR ( 'NONE', #9637, 1000.000000000000000 ) ;
#1807=CIRCLE ( 'NONE', #18754, 0.5079999999999985638 ) ;
#1808=AXIS2_PLACEMENT_3D ( 'NONE', #10508, #6965, #15505 ) ;
#1811=EDGE_CURVE ( 'NONE', #7476, #17693, #13183, .T. ) ;
#1816=EDGE_CURVE ( 'NONE', #6920, #19435, #12114, .T. ) ;
#1819=VERTEX_POINT ( 'NONE', #20194 ) ;
#1822=AXIS2_PLACEMENT_3D ( 'NONE', #12937, #19751, #16572 ) ;
#1823=ORIENTED_EDGE ( 'NONE', *, *, #16213, .F. ) ;
#1828=CARTESIAN_POINT ( 'NONE',  ( 38.96848998618624904, -7.547609999999999708, -3.934807454472129429 ) ) ;
#1833=EDGE_CURVE ( 'NONE', #8981, #14185, #11815, .T. ) ;
#1834=EDGE_CURVE ( 'NONE', #7504, #3737, #15369, .T. ) ;
#1842=VECTOR ( 'NONE', #10307, 1000.000000000000000 ) ;
#1848=CIRCLE ( 'NONE', #9980, 1.190625000000000711 ) ;
#1849=ORIENTED_EDGE ( 'NONE', *, *, #11024, .F. ) ;
#1850=CARTESIAN_POINT ( 'NONE',  ( 61.81956123787853130, 32.54502000000000095, -1.238102447480925239 ) ) ;
#1853=DIRECTION ( 'NONE',  ( 0.000000000000000000, -1.000000000000000000, -0.000000000000000000 ) ) ;
#1867=AXIS2_PLACEMENT_3D ( 'NONE', #3956, #8024, #7701 ) ;
#1868=CARTESIAN_POINT ( 'NONE',  ( 54.55586098912687731, -1.983739999999999837, -6.056925149195119040 ) ) ;
#1873=CARTESIAN_POINT ( 'NONE',  ( 61.02111788801703085, 0.000000000000000000, -5.406220493519755088 ) ) ;
#1879=CARTESIAN_POINT ( 'NONE',  ( 39.07078961959606289, -1.983739999999999837, -27.14892015257980162 ) ) ;
#1881=ORIENTED_EDGE ( 'NONE', *, *, #4165, .T. ) ;
#1887=FACE_OUTER_BOUND ( 'NONE', #6145, .T. ) ;
#1889=AXIS2_PLACEMENT_3D ( 'NONE', #2423, #7065, #12269 ) ;
#1890=DIRECTION ( 'NONE',  ( 0.2064631973582987667, 0.000000000000000000, -0.9784543669157944601 ) ) ;
#1901=CYLINDRICAL_SURFACE ( 'NONE', #4345, 0.5080000000000023386 ) ;
#1913=PLANE ( 'NONE',  #18047 ) ;
#1914=CARTESIAN_POINT ( 'NONE',  ( 54.55586098912687731, -9.531985000000000596, -6.056925149195119040 ) ) ;
#1915=DIRECTION ( 'NONE',  ( 0.05085730733808393328, 0.000000000000000000, -0.9987059298363656357 ) ) ;
#1916=AXIS2_PLACEMENT_3D ( 'NONE', #7858, #11283, #4544 ) ;
#1923=CYLINDRICAL_SURFACE ( 'NONE', #18506, 0.7950200000000003930 ) ;
#1926=UNCERTAINTY_MEASURE_WITH_UNIT (LENGTH_MEASURE( 1.000000000000000082E-05 ), #12674, 'distance_accuracy_value', 'NONE');
#1927=CARTESIAN_POINT ( 'NONE',  ( 52.96420052373725440, 0.000000000000000000, 7.017842122255405712 ) ) ;
#1933=CARTESIAN_POINT ( 'NONE',  ( 46.03750000000000142, 42.06303499999999929, -10.31874999999999964 ) ) ;
#1940=EDGE_LOOP ( 'NONE', ( #14741, #1746, #6135, #11189 ) ) ;
#1941=DIRECTION ( 'NONE',  ( 0.000000000000000000, 1.000000000000000000, 0.000000000000000000 ) ) ;
#1942=ORIENTED_EDGE ( 'NONE', *, *, #3071, .T. ) ;
#1946=FACE_OUTER_BOUND ( 'NONE', #5301, .T. ) ;
#1947=DIRECTION ( 'NONE',  ( 0.000000000000000000, -1.000000000000000000, -0.000000000000000000 ) ) ;
#1948=EDGE_CURVE ( 'NONE', #17792, #1329, #7039, .T. ) ;
#1949=LINE ( 'NONE', #11588, #21721 ) ;
#1951=EDGE_CURVE ( 'NONE', #19608, #17559, #9133, .T. ) ;
#1955=CARTESIAN_POINT ( 'NONE',  ( 38.82016491058538321, 34.52875999999999834, -14.75770094105646812 ) ) ;
#1965=DIRECTION ( 'NONE',  ( 0.000000000000000000, -1.000000000000000000, -0.000000000000000000 ) ) ;
#1966=VERTEX_POINT ( 'NONE', #15473 ) ;
#1969=CARTESIAN_POINT ( 'NONE',  ( 60.38511073144201191, -1.983739999999999837, -22.26373525985038526 ) ) ;
#1970=EDGE_LOOP ( 'NONE', ( #13062, #3651, #5071, #11243 ) ) ;
#1973=ORIENTED_EDGE ( 'NONE', *, *, #9073, .T. ) ;
#1976=CARTESIAN_POINT ( 'NONE',  ( 59.55063415577301811, 34.52875999999999834, -22.52230776719629191 ) ) ;
#1983=DIRECTION ( 'NONE',  ( -0.6702301885068632226, 0.000000000000000000, -0.7421532822901576454 ) ) ;
#1984=CARTESIAN_POINT ( 'NONE',  ( 52.89469146228504570, -5.197312526642835273, -16.93126689015821640 ) ) ;
#1990=VERTEX_POINT ( 'NONE', #525 ) ;
#1992=DIRECTION ( 'NONE',  ( 0.2227372614607789347, 0.000000000000000000, 0.9748785115884710528 ) ) ;
#1998=VECTOR ( 'NONE', #9440, 1000.000000000000000 ) ;
#2003=CARTESIAN_POINT ( 'NONE',  ( 38.23013820809905638, 109.3223030719999969, -14.22485453658974031 ) ) ;
#2008=DIRECTION ( 'NONE',  ( 0.6702301885068638887, 0.000000000000000000, 0.7421532822901570903 ) ) ;
#2010=DIRECTION ( 'NONE',  ( 0.7421532822901569793, 0.000000000000000000, -0.6702301885068642218 ) ) ;
#2014=ORIENTED_EDGE ( 'NONE', *, *, #1415, .F. ) ;
#2016=DIRECTION ( 'NONE',  ( 0.000000000000000000, 1.000000000000000000, 0.000000000000000000 ) ) ;
#2018=B_SPLINE_CURVE_WITH_KNOTS ( 'NONE', 3,
 ( #546, #8824, #7189, #18994, #3871, #10608, #17357, #8941, #14712, #1198 ),
 .UNSPECIFIED., .F., .F.,
 ( 4, 2, 2, 2, 4 ),
 ( 0.006416468533192019007, 0.006892176379334203663, 0.007367884225476389187, 0.007843592071618573844, 0.008319299917760758500 ),
 .UNSPECIFIED. ) ;
#2025=EDGE_CURVE ( 'NONE', #1512, #9499, #10357, .T. ) ;
#2026=AXIS2_PLACEMENT_3D ( 'NONE', #18346, #3213, #1549 ) ;
#2030=VERTEX_POINT ( 'NONE', #12359 ) ;
#2043=ADVANCED_FACE ( 'NONE', ( #19085 ), #17446, .F. ) ;
#2046=ORIENTED_EDGE ( 'NONE', *, *, #21118, .T. ) ;
#2049=ADVANCED_FACE ( 'NONE', ( #1284 ), #11349, .T. ) ;
#2052=CARTESIAN_POINT ( 'NONE',  ( 55.27198911326564001, 0.000000000000000000, 2.462719476673013830 ) ) ;
#2058=DIRECTION ( 'NONE',  ( 0.000000000000000000, -1.000000000000000000, -0.000000000000000000 ) ) ;
#2059=CYLINDRICAL_SURFACE ( 'NONE', #20534, 30.16249999999999076 ) ;
#2071=ORIENTED_EDGE ( 'NONE', *, *, #14354, .F. ) ;
#2072=ORIENTED_EDGE ( 'NONE', *, *, #14472, .F. ) ;
#2083=DIRECTION ( 'NONE',  ( -0.7421532822901579785, 0.000000000000000000, 0.6702301885068628895 ) ) ;
#2084=DIRECTION ( 'NONE',  ( 0.4987171968201928873, 0.000000000000000000, -0.8667647648559606566 ) ) ;
#2085=FACE_OUTER_BOUND ( 'NONE', #10972, .T. ) ;
#2096=VERTEX_POINT ( 'NONE', #9357 ) ;
#2101=CARTESIAN_POINT ( 'NONE',  ( 49.79678389823170903, 0.000000000000000000, -28.13445659451038594 ) ) ;
#2104=VECTOR ( 'NONE', #791, 1000.000000000000114 ) ;
#2110=AXIS2_PLACEMENT_3D ( 'NONE', #16637, #18498, #12100 ) ;
#2117=CIRCLE ( 'NONE', #12729, 1.190625000000000711 ) ;
#2120=CYLINDRICAL_SURFACE ( 'NONE', #3730, 0.5079999999999984528 ) ;
#2128=CARTESIAN_POINT ( 'NONE',  ( 61.83151161312219557, 34.52875999999999834, -0.3645647634491749334 ) ) ;
#2133=ADVANCED_FACE ( 'NONE', ( #19849 ), #953, .F. ) ;
#2135=CARTESIAN_POINT ( 'NONE',  ( 52.91483696501514800, -5.165959288209053923, -16.50498455623153404 ) ) ;
#2150=FACE_OUTER_BOUND ( 'NONE', #12578, .T. ) ;
#2153=PLANE ( 'NONE',  #1078 ) ;
#2156=CARTESIAN_POINT ( 'NONE',  ( 35.15748561355322011, 0.000000000000000000, 0.3244898641346534163 ) ) ;
#2161=FACE_OUTER_BOUND ( 'NONE', #5062, .T. ) ;
#2162=ORIENTED_EDGE ( 'NONE', *, *, #21483, .F. ) ;
#2163=VECTOR ( 'NONE', #13334, 1000.000000000000114 ) ;
#2164=DIRECTION ( 'NONE',  ( 0.2064631973582987667, 0.000000000000000000, -0.9784543669157944601 ) ) ;
#2166=FACE_OUTER_BOUND ( 'NONE', #10801, .T. ) ;
#2169=VECTOR ( 'NONE', #11187, 1000.000000000000114 ) ;
#2171=VECTOR ( 'NONE', #10766, 1000.000000000000000 ) ;
#2172=FACE_OUTER_BOUND ( 'NONE', #5735, .T. ) ;
#2174=CIRCLE ( 'NONE', #3588, 1.190625000000000711 ) ;
#2176=ORIENTED_EDGE ( 'NONE', *, *, #12352, .F. ) ;
#2189=ORIENTED_EDGE ( 'NONE', *, *, #10352, .F. ) ;
#2193=EDGE_CURVE ( 'NONE', #10898, #10146, #855, .T. ) ;
#2195=ADVANCED_FACE ( 'NONE', ( #19411 ), #12809, .T. ) ;
#2197=VECTOR ( 'NONE', #14140, 1000.000000000000000 ) ;
#2198=ORIENTED_EDGE ( 'NONE', *, *, #9674, .F. ) ;
#2202=DIRECTION ( 'NONE',  ( 0.000000000000000000, 1.000000000000000000, 0.000000000000000000 ) ) ;
#2206=CARTESIAN_POINT ( 'NONE',  ( 46.03750000000000142, -9.531985000000000596, -10.31874999999999964 ) ) ;
#2209=DIRECTION ( 'NONE',  ( 0.000000000000000000, -1.000000000000000000, -0.000000000000000000 ) ) ;
#2210=VECTOR ( 'NONE', #20023, 1000.000000000000000 ) ;
#2211=ORIENTED_EDGE ( 'NONE', *, *, #20541, .T. ) ;
#2227=VECTOR ( 'NONE', #21862, 1000.000000000000000 ) ;
#2234=AXIS2_PLACEMENT_3D ( 'NONE', #14022, #2275, #17644 ) ;
#2248=VERTEX_POINT ( 'NONE', #14984 ) ;
#2251=CIRCLE ( 'NONE', #18482, 0.5080000000000005622 ) ;
#2257=AXIS2_PLACEMENT_3D ( 'NONE', #14167, #7396, #12497 ) ;
#2259=CARTESIAN_POINT ( 'NONE',  ( 42.35466991749225940, 0.000000000000000000, -17.94967221382040279 ) ) ;
#2264=ORIENTED_EDGE ( 'NONE', *, *, #18406, .F. ) ;
#2267=DIRECTION ( 'NONE',  ( 0.000000000000000000, 1.000000000000000000, 0.000000000000000000 ) ) ;
#2268=ORIENTED_EDGE ( 'NONE', *, *, #13671, .F. ) ;
#2274=ORIENTED_EDGE ( 'NONE', *, *, #4323, .F. ) ;
#2275=DIRECTION ( 'NONE',  ( 0.000000000000000000, 0.000000000000000000, 1.000000000000000000 ) ) ;
#2276=VECTOR ( 'NONE', #11207, 1000.000000000000000 ) ;
#2278=EDGE_LOOP ( 'NONE', ( #17666, #4526, #8474, #2014, #7296, #13122 ) ) ;
#2279=DIRECTION ( 'NONE',  ( 0.05085730733808142834, 0.000000000000000000, -0.9987059298363657467 ) ) ;
#2282=CARTESIAN_POINT ( 'NONE',  ( 52.19854938732527216, 38.88803500000000213, -17.58284632693144189 ) ) ;
#2284=VECTOR ( 'NONE', #16090, 1000.000000000000000 ) ;
#2290=ORIENTED_EDGE ( 'NONE', *, *, #4296, .T. ) ;
#2295=ORIENTED_EDGE ( 'NONE', *, *, #2372, .F. ) ;
#2302=VERTEX_POINT ( 'NONE', #21585 ) ;
#2303=AXIS2_PLACEMENT_3D ( 'NONE', #6826, #18541, #18638 ) ;
#2312=EDGE_CURVE ( 'NONE', #10134, #7286, #8239, .T. ) ;
#2313=CARTESIAN_POINT ( 'NONE',  ( 53.45144661199496028, 38.88803500000000213, -15.40991637425222827 ) ) ;
#2320=CYLINDRICAL_SURFACE ( 'NONE', #2800, 30.16250000000000142 ) ;
#2321=ORIENTED_EDGE ( 'NONE', *, *, #10762, .F. ) ;
#2331=CARTESIAN_POINT ( 'NONE',  ( 47.80475250345343596, -7.547610000000002373, -11.91473563638196786 ) ) ;
#2332=LINE ( 'NONE', #5862, #1679 ) ;
#2335=CYLINDRICAL_SURFACE ( 'NONE', #15678, 1.190625000000000488 ) ;
#2339=CARTESIAN_POINT ( 'NONE',  ( 32.55306802826559220, 0.000000000000000000, -17.37731658638881527 ) ) ;
#2348=DIRECTION ( 'NONE',  ( 0.000000000000000000, 1.000000000000000000, 0.000000000000000000 ) ) ;
#2351=DIRECTION ( 'NONE',  ( -0.1060008583745199739, 0.000000000000000000, -0.9943660382494290406 ) ) ;
#2354=CARTESIAN_POINT ( 'NONE',  ( 49.13030338002142372, -9.531985000000000596, -2.154981381712871791 ) ) ;
#2359=ORIENTED_EDGE ( 'NONE', *, *, #4471, .T. ) ;
#2361=FACE_OUTER_BOUND ( 'NONE', #13362, .T. ) ;
#2365=EDGE_CURVE ( 'NONE', #1425, #17778, #19192, .T. ) ;
#2372=EDGE_CURVE ( 'NONE', #1209, #19005, #10519, .T. ) ;
#2373=CARTESIAN_POINT ( 'NONE',  ( 61.04701390398659555, 0.000000000000000000, -15.15157976445104993 ) ) ;
#2375=LINE ( 'NONE', #20819, #10264 ) ;
#2387=ORIENTED_EDGE ( 'NONE', *, *, #13897, .T. ) ;
#2391=ORIENTED_EDGE ( 'NONE', *, *, #11011, .F. ) ;
#2395=EDGE_CURVE ( 'NONE', #3338, #7171, #493, .T. ) ;
#2396=VECTOR ( 'NONE', #17884, 1000.000000000000000 ) ;
#2398=ORIENTED_EDGE ( 'NONE', *, *, #18799, .T. ) ;
#2399=CARTESIAN_POINT ( 'NONE',  ( 53.25483508941461963, 0.000000000000000000, -5.879799058943532941 ) ) ;
#2400=LINE ( 'NONE', #4392, #3205 ) ;
#2403=CARTESIAN_POINT ( 'NONE',  ( 38.96521490655496223, -7.547609999999999708, -3.938433986281342225 ) ) ;
#2404=ORIENTED_EDGE ( 'NONE', *, *, #11133, .T. ) ;
#2405=DIRECTION ( 'NONE',  ( 0.6702301885068628895, 0.000000000000000000, 0.7421532822901579785 ) ) ;
#2418=ADVANCED_FACE ( 'NONE', ( #7320 ), #12295, .F. ) ;
#2419=ORIENTED_EDGE ( 'NONE', *, *, #1951, .F. ) ;
#2421=VECTOR ( 'NONE', #18715, 1000.000000000000114 ) ;
#2423=CARTESIAN_POINT ( 'NONE',  ( 31.02798609601340729, 0.000000000000000000, -5.485920235548950252 ) ) ;
#2424=CARTESIAN_POINT ( 'NONE',  ( 61.56621290189396944, -1.983739999999999837, -0.7977859469341201937 ) ) ;
#2426=CARTESIAN_POINT ( 'NONE',  ( 55.27198911326564001, 32.54502000000000095, 2.462719476673013830 ) ) ;
#2433=PLANE ( 'NONE',  #789 ) ;
#2437=DIRECTION ( 'NONE',  ( 0.000000000000000000, -1.000000000000000000, -0.000000000000000000 ) ) ;
#2440=ORIENTED_EDGE ( 'NONE', *, *, #8438, .T. ) ;
#2442=LINE ( 'NONE', #10945, #6725 ) ;
#2446=CYLINDRICAL_SURFACE ( 'NONE', #1340, 0.5079999999999996740 ) ;
#2450=CARTESIAN_POINT ( 'NONE',  ( 59.89111109153450485, 29.95901653600000003, -22.14529389979288965 ) ) ;
#2452=DIRECTION ( 'NONE',  ( -0.9987059298363656357, 0.000000000000000000, -0.05085730733808393328 ) ) ;
#2455=CIRCLE ( 'NONE', #13065, 30.16249999999998366 ) ;
#2456=PLANE ( 'NONE',  #1174 ) ;
#2458=CARTESIAN_POINT ( 'NONE',  ( 30.47347900023190803, 32.54502000000000095, -8.148724574017967015 ) ) ;
#2462=CARTESIAN_POINT ( 'NONE',  ( 59.80894853325292360, -6.356984999999999886, -16.70545285374888778 ) ) ;
#2469=CARTESIAN_POINT ( 'NONE',  ( 30.41963056417667488, 32.54502000000000095, -8.653862521447852174 ) ) ;
#2470=EDGE_LOOP ( 'NONE', ( #5241, #5173 ) ) ;
#2476=ORIENTED_EDGE ( 'NONE', *, *, #19653, .F. ) ;
#2478=VECTOR ( 'NONE', #10363, 1000.000000000000000 ) ;
#2479=CIRCLE ( 'NONE', #14857, 30.16249999999999432 ) ;
#2481=DIRECTION ( 'NONE',  ( 0.000000000000000000, -1.000000000000000000, -0.000000000000000000 ) ) ;
#2483=DIRECTION ( 'NONE',  ( 0.000000000000000000, -1.000000000000000000, 0.000000000000000000 ) ) ;
#2488=CARTESIAN_POINT ( 'NONE',  ( 52.19854938732527216, 39.04666396067986511, -17.58284632693144189 ) ) ;
#2494=FACE_OUTER_BOUND ( 'NONE', #2970, .T. ) ;
#2497=CARTESIAN_POINT ( 'NONE',  ( 39.79827138724637337, -6.045821519594339222, -3.121440830586406090 ) ) ;
#2499=ADVANCED_FACE ( 'NONE', ( #7643 ), #21337, .F. ) ;
#2509=VERTEX_POINT ( 'NONE', #21230 ) ;
#2511=EDGE_CURVE ( 'NONE', #7874, #13814, #4187, .T. ) ;
#2515=ORIENTED_EDGE ( 'NONE', *, *, #3919, .F. ) ;
#2524=VERTEX_POINT ( 'NONE', #13073 ) ;
#2527=ORIENTED_EDGE ( 'NONE', *, *, #11249, .F. ) ;
#2528=ORIENTED_EDGE ( 'NONE', *, *, #5424, .F. ) ;
#2529=VECTOR ( 'NONE', #15760, 1000.000000000000000 ) ;
#2530=VECTOR ( 'NONE', #16813, 1000.000000000000000 ) ;
#2535=CARTESIAN_POINT ( 'NONE',  ( 54.61912012054379062, -6.356984999999999886, -13.79062155615056362 ) ) ;
#2539=CARTESIAN_POINT ( 'NONE',  ( 61.09555596642878328, 34.52875999999999834, -12.53419992421059348 ) ) ;
#2544=ORIENTED_EDGE ( 'NONE', *, *, #10432, .T. ) ;
#2547=CARTESIAN_POINT ( 'NONE',  ( 57.35354854712898742, -1.983739999999999837, -21.22263945788050776 ) ) ;
#2550=AXIS2_PLACEMENT_3D ( 'NONE', #7940, #4741, #2645 ) ;
#2556=CARTESIAN_POINT ( 'NONE',  ( 27.87822510359947614, 37.11476346399999926, -8.893823290944665061 ) ) ;
#2560=CARTESIAN_POINT ( 'NONE',  ( 45.06824031473712466, -6.356984999999999886, -7.839138111891783112 ) ) ;
#2562=DIRECTION ( 'NONE',  ( 0.000000000000000000, -1.000000000000000000, -0.000000000000000000 ) ) ;
#2567=CARTESIAN_POINT ( 'NONE',  ( 38.82016491058538321, 0.000000000000000000, -14.75770094105646812 ) ) ;
#2572=ORIENTED_EDGE ( 'NONE', *, *, #14972, .F. ) ;
#2583=VERTEX_POINT ( 'NONE', #1868 ) ;
#2587=VERTEX_POINT ( 'NONE', #19994 ) ;
#2593=CARTESIAN_POINT ( 'NONE',  ( 53.25207718670083779, -7.553614316632189407, -16.53988246642675009 ) ) ;
#2597=DIRECTION ( 'NONE',  ( -0.9943660382494290406, 0.000000000000000000, 0.1060008583745199739 ) ) ;
#2599=VERTEX_POINT ( 'NONE', #4967 ) ;
#2600=EDGE_CURVE ( 'NONE', #12951, #7504, #7908, .T. ) ;
#2608=DIRECTION ( 'NONE',  ( -0.000000000000000000, -1.000000000000000000, 0.000000000000000000 ) ) ;
#2610=SHAPE_REPRESENTATION_RELATIONSHIP ( 'NONE' , 'NONE' ,  #3526, #6907 ) ;
#2612=CARTESIAN_POINT ( 'NONE',  ( 31.02798609601340729, 0.000000000000000000, -5.485920235548950252 ) ) ;
#2625=VERTEX_POINT ( 'NONE', #11609 ) ;
#2631=EDGE_LOOP ( 'NONE', ( #6751, #20403, #16132, #5835 ) ) ;
#2640=B_SPLINE_CURVE_WITH_KNOTS ( 'NONE', 3,
 ( #11793, #18526, #3391, #14017, #9009 ),
 .UNSPECIFIED., .F., .F.,
 ( 4, 1, 4 ),
 ( 0.003699823995551414398, 0.003727086906962521692, 0.003754349818373628987 ),
 .UNSPECIFIED. ) ;
#2644=TOROIDAL_SURFACE ( 'NONE', #4064, 3.174999999999999822, 1.190625000000000044 ) ;
#2645=DIRECTION ( 'NONE',  ( 0.6702301885068632226, 0.000000000000000000, 0.7421532822901576454 ) ) ;
#2648=DIRECTION ( 'NONE',  ( 0.2227372614607789347, 0.000000000000000000, 0.9748785115884710528 ) ) ;
#2650=ORIENTED_EDGE ( 'NONE', *, *, #6027, .T. ) ;
#2652=CARTESIAN_POINT ( 'NONE',  ( 49.28028498622276032, 32.54502000000000095, -25.68670502218146368 ) ) ;
#2654=DIRECTION ( 'NONE',  ( 0.000000000000000000, -1.000000000000000000, -0.000000000000000000 ) ) ;
#2655=CARTESIAN_POINT ( 'NONE',  ( 42.27821610176829381, 32.54502000000000095, 7.496956594510385763 ) ) ;
#2656=ORIENTED_EDGE ( 'NONE', *, *, #1137, .F. ) ;
#2659=LINE ( 'NONE', #18016, #14030 ) ;
#2660=CARTESIAN_POINT ( 'NONE',  ( 39.16413618835606769, 0.000000000000000000, -24.45043885672975392 ) ) ;
#2662=EDGE_LOOP ( 'NONE', ( #6177, #3400, #13676, #18605 ) ) ;
#2664=ORIENTED_EDGE ( 'NONE', *, *, #21131, .F. ) ;
#2665=PLANE ( 'NONE',  #14862 ) ;
#2669=CARTESIAN_POINT ( 'NONE',  ( 55.27198911326564001, 0.000000000000000000, 2.462719476673013830 ) ) ;
#2671=ADVANCED_FACE ( 'NONE', ( #18663 ), #10160, .F. ) ;
#2673=B_SPLINE_CURVE_WITH_KNOTS ( 'NONE', 3,
 ( #19929, #11532, #7994, #19704 ),
 .UNSPECIFIED., .F., .F.,
 ( 4, 4 ),
 ( -7.968845587668896464E-05, 0.0005317181549816462575 ),
 .UNSPECIFIED. ) ;
#2674=AXIS2_PLACEMENT_3D ( 'NONE', #14768, #6332, #21592 ) ;
#2677=DIRECTION ( 'NONE',  ( 0.000000000000000000, 1.000000000000000000, 0.000000000000000000 ) ) ;
#2689=CARTESIAN_POINT ( 'NONE',  ( 53.25483508941461963, -9.531985000000000596, -5.879799058943532941 ) ) ;
#2704=DIRECTION ( 'NONE',  ( -0.9959941601142525691, 0.000000000000000000, -0.08941830359777946935 ) ) ;
#2705=VERTEX_POINT ( 'NONE', #15388 ) ;
#2717=FACE_OUTER_BOUND ( 'NONE', #21076, .T. ) ;
#2726=CIRCLE ( 'NONE', #14759, 1.190624999999997824 ) ;
#2727=FACE_OUTER_BOUND ( 'NONE', #524, .T. ) ;
#2728=ORIENTED_EDGE ( 'NONE', *, *, #10631, .T. ) ;
#2735=CARTESIAN_POINT ( 'NONE',  ( 61.81956123787853130, -1.983739999999999837, -1.238102447480925239 ) ) ;
#2738=EDGE_CURVE ( 'NONE', #19531, #3414, #6496, .T. ) ;
#2740=AXIS2_PLACEMENT_3D ( 'NONE', #1315, #13281, #15050 ) ;
#2742=EDGE_CURVE ( 'NONE', #2587, #5690, #11932, .T. ) ;
#2744=EDGE_CURVE ( 'NONE', #10152, #13027, #2977, .T. ) ;
#2749=CARTESIAN_POINT ( 'NONE',  ( 30.41963056417667488, 34.52875999999999834, -8.653862521447852174 ) ) ;
#2758=EDGE_LOOP ( 'NONE', ( #819, #5356, #9094, #1296 ) ) ;
#2784=PLANE ( 'NONE',  #9934 ) ;
#2785=AXIS2_PLACEMENT_3D ( 'NONE', #5633, #2209, #12059 ) ;
#2797=DIRECTION ( 'NONE',  ( 0.000000000000000000, 1.000000000000000000, 0.000000000000000000 ) ) ;
#2800=AXIS2_PLACEMENT_3D ( 'NONE', #770, #17474, #9053 ) ;
#2801=DIRECTION ( 'NONE',  ( 0.7421532822901579785, 0.000000000000000000, -0.6702301885068628895 ) ) ;
#2805=VECTOR ( 'NONE', #6594, 1000.000000000000000 ) ;
#2807=DIRECTION ( 'NONE',  ( 0.000000000000000000, 1.000000000000000000, 0.000000000000000000 ) ) ;
#2809=AXIS2_PLACEMENT_3D ( 'NONE', #8306, #1241, #18362 ) ;
#2816=EDGE_CURVE ( 'NONE', #8109, #11708, #15601, .T. ) ;
#2824=LINE ( 'NONE', #1370, #15156 ) ;
#2836=ORIENTED_EDGE ( 'NONE', *, *, #21101, .T. ) ;
#2846=DIRECTION ( 'NONE',  ( 0.3542738219355897056, 0.000000000000000000, 0.9351417320872542627 ) ) ;
#2849=ORIENTED_EDGE ( 'NONE', *, *, #4636, .T. ) ;
#2854=AXIS2_PLACEMENT_3D ( 'NONE', #11762, #13536, #10529 ) ;
#2863=ORIENTED_EDGE ( 'NONE', *, *, #3055, .T. ) ;
#2867=DIRECTION ( 'NONE',  ( -0.07875956036501312318, 0.000000000000000000, 0.9968936410927243807 ) ) ;
#2870=EDGE_LOOP ( 'NONE', ( #14960, #15454, #8532, #8925 ) ) ;
#2872=EDGE_CURVE ( 'NONE', #12131, #20877, #1197, .T. ) ;
#2874=EDGE_CURVE ( 'NONE', #5388, #3524, #19220, .T. ) ;
#2876=DIRECTION ( 'NONE',  ( 0.000000000000000000, -1.000000000000000000, -0.000000000000000000 ) ) ;
#2878=ORIENTED_EDGE ( 'NONE', *, *, #1009, .T. ) ;
#2879=AXIS2_PLACEMENT_3D ( 'NONE', #584, #4344, #8978 ) ;
#2880=ORIENTED_EDGE ( 'NONE', *, *, #13843, .T. ) ;
#2881=DIRECTION ( 'NONE',  ( 0.000000000000000000, 1.000000000000000000, 0.000000000000000000 ) ) ;
#2884=CIRCLE ( 'NONE', #1465, 1.190625000000000711 ) ;
#2885=CIRCLE ( 'NONE', #21227, 1.190625000000000711 ) ;
#2899=CIRCLE ( 'NONE', #15272, 1.190625000000000711 ) ;
#2901=EDGE_CURVE ( 'NONE', #119, #2583, #8256, .T. ) ;
#2904=DIRECTION ( 'NONE',  ( 0.000000000000000000, -1.000000000000000000, -0.000000000000000000 ) ) ;
#2908=AXIS2_PLACEMENT_3D ( 'NONE', #10400, #4976, #1760 ) ;
#2909=CYLINDRICAL_SURFACE ( 'NONE', #8787, 30.16250000000000497 ) ;
#2911=CARTESIAN_POINT ( 'NONE',  ( 61.04701390398659555, 32.54502000000000095, -15.15157976445104993 ) ) ;
#2914=DIRECTION ( 'NONE',  ( 0.000000000000000000, 1.000000000000000000, 0.000000000000000000 ) ) ;
#2919=EDGE_CURVE ( 'NONE', #1535, #2096, #11089, .T. ) ;
#2925=EDGE_CURVE ( 'NONE', #11597, #16209, #11437, .T. ) ;
#2926=VECTOR ( 'NONE', #5481, 1000.000000000000000 ) ;
#2927=CARTESIAN_POINT ( 'NONE',  ( 53.25483508941461963, -9.531985000000000596, -5.879799058943532941 ) ) ;
#2938=LINE ( 'NONE', #6235, #6329 ) ;
#2940=CYLINDRICAL_SURFACE ( 'NONE', #15959, 9.524999999999998579 ) ;
#2945=CARTESIAN_POINT ( 'NONE',  ( 45.06824031473797021, 38.88803500000000213, -7.839138111890849636 ) ) ;
#2953=EDGE_CURVE ( 'NONE', #16343, #6924, #2018, .T. ) ;
#2956=FILL_AREA_STYLE ('',( #10012 ) ) ;
#2966=ORIENTED_EDGE ( 'NONE', *, *, #19024, .F. ) ;
#2970=EDGE_LOOP ( 'NONE', ( #17589, #15029, #9937, #142, #13916, #19267 ) ) ;
#2977=CIRCLE ( 'NONE', #18834, 1.190624999999997824 ) ;
#2978=LINE ( 'NONE', #11254, #7567 ) ;
#2980=DIRECTION ( 'NONE',  ( 0.05085730733808393328, 0.000000000000000000, -0.9987059298363656357 ) ) ;
#2985=DIRECTION ( 'NONE',  ( 0.000000000000000000, 1.000000000000000000, 0.000000000000000000 ) ) ;
#2986=DIRECTION ( 'NONE',  ( 0.000000000000000000, 1.000000000000000000, 0.000000000000000000 ) ) ;
#2987=CARTESIAN_POINT ( 'NONE',  ( 56.91751438644678984, 0.000000000000000000, -20.96198986413465448 ) ) ;
#2992=CIRCLE ( 'NONE', #15356, 0.5079999999999976756 ) ;
#3016=ORIENTED_EDGE ( 'NONE', *, *, #3725, .T. ) ;
#3018=DIRECTION ( 'NONE',  ( -0.6702301885068630005, 0.000000000000000000, -0.7421532822901579785 ) ) ;
#3021=CARTESIAN_POINT ( 'NONE',  ( 49.41195815393805901, 42.06303499999999929, -1.411525001868561224 ) ) ;
#3028=EDGE_CURVE ( 'NONE', #7335, #17408, #19956, .T. ) ;
#3031=PLANE ( 'NONE',  #17410 ) ;
#3032=CARTESIAN_POINT ( 'NONE',  ( 53.92979111630407374, -6.356984999999459873, -15.65141968182990162 ) ) ;
#3033=CYLINDRICAL_SURFACE ( 'NONE', #2674, 1.190624999999999378 ) ;
#3041=CARTESIAN_POINT ( 'NONE',  ( 52.76334005444670794, 38.88803500000000213, -23.57731578991186083 ) ) ;
#3045=DIRECTION ( 'NONE',  ( -0.6702301885068630005, 0.000000000000000000, -0.7421532822901579785 ) ) ;
#3049=CARTESIAN_POINT ( 'NONE',  ( 46.03750000000000142, -9.531985000000000596, -10.31874999999999964 ) ) ;
#3055=EDGE_CURVE ( 'NONE', #14160, #18035, #18119, .T. ) ;
#3056=CARTESIAN_POINT ( 'NONE',  ( 38.22597429223493748, 39.04395605175655248, -4.868457244536984696 ) ) ;
#3060=ORIENTED_EDGE ( 'NONE', *, *, #21551, .T. ) ;
#3063=LINE ( 'NONE', #1181, #3943 ) ;
#3068=CARTESIAN_POINT ( 'NONE',  ( 46.03750000000000142, -1.983739999999999837, -10.31874999999999964 ) ) ;
#3069=ORIENTED_EDGE ( 'NONE', *, *, #6085, .T. ) ;
#3071=EDGE_CURVE ( 'NONE', #8830, #13930, #2978, .T. ) ;
#3072=ORIENTED_EDGE ( 'NONE', *, *, #12490, .F. ) ;
#3073=ADVANCED_FACE ( 'NONE', ( #970 ), #16468, .F. ) ;
#3081=DIRECTION ( 'NONE',  ( 0.000000000000000000, 1.000000000000000000, 0.000000000000000000 ) ) ;
#3082=CARTESIAN_POINT ( 'NONE',  ( 32.42378190387104553, 34.52875999999999834, -18.15178106273469183 ) ) ;
#3085=EDGE_LOOP ( 'NONE', ( #12373, #15790, #10238, #21050 ) ) ;
#3086=CYLINDRICAL_SURFACE ( 'NONE', #19163, 0.5080000000000023386 ) ;
#3087=CARTESIAN_POINT ( 'NONE',  ( 32.17043356788648367, 32.54502000000000095, -17.71146456218788146 ) ) ;
#3089=CARTESIAN_POINT ( 'NONE',  ( 53.83137747314165722, 38.57687151959435568, -15.79457933408115089 ) ) ;
#3090=ORIENTED_EDGE ( 'NONE', *, *, #5055, .F. ) ;
#3091=VERTEX_POINT ( 'NONE', #19551 ) ;
#3094=DIRECTION ( 'NONE',  ( -0.9987059298363657467, 0.000000000000000000, -0.05085730733808409287 ) ) ;
#3095=VERTEX_POINT ( 'NONE', #4418 ) ;
#3098=PLANE ( 'NONE',  #8140 ) ;
#3100=AXIS2_PLACEMENT_3D ( 'NONE', #4172, #6039, #14259 ) ;
#3113=CARTESIAN_POINT ( 'NONE',  ( 37.35186600153178915, 38.88803500000000213, -2.356229033655170113 ) ) ;
#3115=VERTEX_POINT ( 'NONE', #4189 ) ;
#3124=EDGE_LOOP ( 'NONE', ( #11928, #5178, #8186, #2072 ) ) ;
#3125=CARTESIAN_POINT ( 'NONE',  ( 32.18388890846549799, 34.52875999999999834, 1.507793899792891468 ) ) ;
#3129=LINE ( 'NONE', #11636, #5032 ) ;
#3134=CARTESIAN_POINT ( 'NONE',  ( 30.41963056417667488, 32.54502000000000095, -8.653862521447852174 ) ) ;
#3136=LINE ( 'NONE', #16630, #17400 ) ;
#3137=DIRECTION ( 'NONE',  ( -0.3928209820863007296, 0.000000000000000000, 0.9196149607486571176 ) ) ;
#3142=CARTESIAN_POINT ( 'NONE',  ( 46.03750000000000142, -9.531985000000000596, -10.31874999999999964 ) ) ;
#3143=EDGE_CURVE ( 'NONE', #16035, #7874, #18138, .T. ) ;
#3149=LINE ( 'NONE', #21492, #8411 ) ;
#3156=EDGE_CURVE ( 'NONE', #21599, #17693, #18225, .T. ) ;
#3165=LINE ( 'NONE', #9897, #2805 ) ;
#3166=EDGE_CURVE ( 'NONE', #3464, #7494, #8611, .T. ) ;
#3168=LINE ( 'NONE', #16348, #14535 ) ;
#3173=VERTEX_POINT ( 'NONE', #17080 ) ;
#3180=AXIS2_PLACEMENT_3D ( 'NONE', #19584, #21237, #19469 ) ;
#3184=CARTESIAN_POINT ( 'NONE',  ( 53.11257091495114935, -7.547610000000002373, -16.69598124282935458 ) ) ;
#3189=VERTEX_POINT ( 'NONE', #8266 ) ;
#3191=LINE ( 'NONE', #13477, #9964 ) ;
#3197=AXIS2_PLACEMENT_3D ( 'NONE', #2911, #5104, #6758 ) ;
#3202=ORIENTED_EDGE ( 'NONE', *, *, #11727, .F. ) ;
#3205=VECTOR ( 'NONE', #21069, 1000.000000000000000 ) ;
#3208=AXIS2_PLACEMENT_3D ( 'NONE', #6263, #10022, #6493 ) ;
#3209=DIRECTION ( 'NONE',  ( 0.05085730733808393328, 0.000000000000000000, -0.9987059298363656357 ) ) ;
#3213=DIRECTION ( 'NONE',  ( 0.000000000000000000, -1.000000000000000000, -0.000000000000000000 ) ) ;
#3214=ORIENTED_EDGE ( 'NONE', *, *, #7590, .F. ) ;
#3216=CARTESIAN_POINT ( 'NONE',  ( 42.94469661997857912, -9.531985000000000596, -18.48251861828712705 ) ) ;
#3219=AXIS2_PLACEMENT_3D ( 'NONE', #4230, #21031, #16082 ) ;
#3234=VECTOR ( 'NONE', #13395, 1000.000000000000000 ) ;
#3241=FACE_OUTER_BOUND ( 'NONE', #21137, .T. ) ;
#3242=ADVANCED_FACE ( 'NONE', ( #11996 ), #1923, .T. ) ;
#3244=CARTESIAN_POINT ( 'NONE',  ( 48.58367710892853353, 0.000000000000000000, -25.32442392637788231 ) ) ;
#3246=CARTESIAN_POINT ( 'NONE',  ( 39.55018955470821140, 39.86562041721325045, -3.343445860290124028 ) ) ;
#3250=ORIENTED_EDGE ( 'NONE', *, *, #18507, .F. ) ;
#3251=CARTESIAN_POINT ( 'NONE',  ( 47.80475250345343596, 42.06303499999999929, -11.91473563638196786 ) ) ;
#3252=AXIS2_PLACEMENT_3D ( 'NONE', #10278, #10170, #10066 ) ;
#3255=ORIENTED_EDGE ( 'NONE', *, *, #3436, .T. ) ;
#3262=EDGE_LOOP ( 'NONE', ( #11490, #3775, #11036, #12402 ) ) ;
#3280=( NAMED_UNIT ( * ) SI_UNIT ( $, .STERADIAN. ) SOLID_ANGLE_UNIT ( ) );
#3285=ORIENTED_EDGE ( 'NONE', *, *, #1514, .T. ) ;
#3286=ORIENTED_EDGE ( 'NONE', *, *, #9816, .F. ) ;
#3296=EDGE_CURVE ( 'NONE', #10564, #3737, #11811, .T. ) ;
#3298=DIRECTION ( 'NONE',  ( 0.7421532822901580895, -0.000000000000000000, -0.6702301885068630005 ) ) ;
#3302=AXIS2_PLACEMENT_3D ( 'NONE', #7216, #8851, #7091 ) ;
#3304=EDGE_CURVE ( 'NONE', #13139, #4078, #5458, .T. ) ;
#3305=FACE_OUTER_BOUND ( 'NONE', #9165, .T. ) ;
#3308=ORIENTED_EDGE ( 'NONE', *, *, #16549, .T. ) ;
#3314=ORIENTED_EDGE ( 'NONE', *, *, #3919, .T. ) ;
#3315=ORIENTED_EDGE ( 'NONE', *, *, #9816, .T. ) ;
#3319=ORIENTED_EDGE ( 'NONE', *, *, #18555, .T. ) ;
#3321=AXIS2_PLACEMENT_3D ( 'NONE', #15568, #20180, #13579 ) ;
#3326=DIRECTION ( 'NONE',  ( 0.000000000000000000, 1.000000000000000000, 0.000000000000000000 ) ) ;
#3329=DIRECTION ( 'NONE',  ( 0.000000000000000000, -1.000000000000000000, -0.000000000000000000 ) ) ;
#3331=ORIENTED_EDGE ( 'NONE', *, *, #14696, .T. ) ;
#3334=DIRECTION ( 'NONE',  ( 0.000000000000000000, 0.000000000000000000, -1.000000000000000000 ) ) ;
#3335=CARTESIAN_POINT ( 'NONE',  ( 52.69088350064333781, -7.396940496609654581, -17.13629674769522282 ) ) ;
#3338=VERTEX_POINT ( 'NONE', #17746 ) ;
#3346=FACE_OUTER_BOUND ( 'NONE', #7256, .T. ) ;
#3347=ADVANCED_FACE ( 'NONE', ( #7673 ), #12323, .T. ) ;
#3350=EDGE_CURVE ( 'NONE', #21216, #18977, #15715, .T. ) ;
#3362=CARTESIAN_POINT ( 'NONE',  ( 39.44573040579900436, 39.95099742452212865, -3.441431441669689395 ) ) ;
#3370=DIRECTION ( 'NONE',  ( -0.1060008583745224581, 0.000000000000000000, -0.9943660382494288186 ) ) ;
#3372=VECTOR ( 'NONE', #13803, 1000.000000000000114 ) ;
#3373=CARTESIAN_POINT ( 'NONE',  ( 46.03750000000000142, -9.531985000000000596, -10.31874999999999964 ) ) ;
#3374=ADVANCED_FACE ( 'NONE', ( #17629 ), #6006, .T. ) ;
#3376=DIRECTION ( 'NONE',  ( 0.000000000000000000, -1.000000000000000000, -0.000000000000000000 ) ) ;
#3380=CARTESIAN_POINT ( 'NONE',  ( 38.57962667713734817, 37.84782743281653694, -4.391981920076847068 ) ) ;
#3388=DIRECTION ( 'NONE',  ( -0.9987059298363657467, 0.000000000000000000, -0.05085730733808445370 ) ) ;
#3391=CARTESIAN_POINT ( 'NONE',  ( 53.12464125271250737, -5.166565464015373976, -16.68257730012009077 ) ) ;
#3397=EDGE_CURVE ( 'NONE', #5196, #8930, #13238, .T. ) ;
#3400=ORIENTED_EDGE ( 'NONE', *, *, #21525, .F. ) ;
#3403=DIRECTION ( 'NONE',  ( 0.000000000000000000, -1.000000000000000000, 0.000000000000000000 ) ) ;
#3410=EDGE_CURVE ( 'NONE', #2524, #14810, #14658, .T. ) ;
#3411=CARTESIAN_POINT ( 'NONE',  ( 46.03750000000000142, 32.54502000000000095, -10.31874999999999964 ) ) ;
#3412=CARTESIAN_POINT ( 'NONE',  ( 52.44708915697334106, 32.54502000000000095, 4.020247972991190188 ) ) ;
#3414=VERTEX_POINT ( 'NONE', #10990 ) ;
#3415=ORIENTED_EDGE ( 'NONE', *, *, #17099, .T. ) ;
#3417=ORIENTED_EDGE ( 'NONE', *, *, #14010, .F. ) ;
#3421=ORIENTED_EDGE ( 'NONE', *, *, #3725, .F. ) ;
#3425=CARTESIAN_POINT ( 'NONE',  ( 59.89111109153450485, -1.983739999999999837, -22.14529389979288965 ) ) ;
#3434=LINE ( 'NONE', #13727, #2530 ) ;
#3436=EDGE_CURVE ( 'NONE', #1617, #13806, #10759, .T. ) ;
#3446=EDGE_CURVE ( 'NONE', #5914, #20066, #19279, .T. ) ;
#3447=CARTESIAN_POINT ( 'NONE',  ( 31.02798609601340729, 34.52875999999999834, -5.485920235548950252 ) ) ;
#3450=DIRECTION ( 'NONE',  ( 0.05085730733808393328, 0.000000000000000000, -0.9987059298363656357 ) ) ;
#3457=DIRECTION ( 'NONE',  ( 0.6702301885068652210, 0.000000000000000000, 0.7421532822901560911 ) ) ;
#3462=EDGE_CURVE ( 'NONE', #7874, #4463, #8363, .T. ) ;
#3463=TOROIDAL_SURFACE ( 'NONE', #633, 3.174999999999999822, 1.190625000000000044 ) ;
#3464=VERTEX_POINT ( 'NONE', #11638 ) ;
#3466=DIRECTION ( 'NONE',  ( 0.05085730733808393328, 0.000000000000000000, -0.9987059298363656357 ) ) ;
#3467=ORIENTED_EDGE ( 'NONE', *, *, #18533, .T. ) ;
#3471=DIRECTION ( 'NONE',  ( 0.9959941601142464629, 0.000000000000000000, 0.08941830359784717908 ) ) ;
#3477=EDGE_LOOP ( 'NONE', ( #9306, #3319, #14708, #12162 ) ) ;
#3489=ORIENTED_EDGE ( 'NONE', *, *, #21038, .F. ) ;
#3490=EDGE_LOOP ( 'NONE', ( #19039, #9864, #62, #20847 ) ) ;
#3491=AXIS2_PLACEMENT_3D ( 'NONE', #16476, #8053, #11819 ) ;
#3495=DIRECTION ( 'NONE',  ( -0.3928209820863007296, 0.000000000000000000, 0.9196149607486571176 ) ) ;
#3496=ORIENTED_EDGE ( 'NONE', *, *, #114, .T. ) ;
#3499=ORIENTED_EDGE ( 'NONE', *, *, #1244, .T. ) ;
#3502=ORIENTED_EDGE ( 'NONE', *, *, #3975, .F. ) ;
#3504=CARTESIAN_POINT ( 'NONE',  ( 61.65536943582333151, 0.000000000000000000, -11.98363747855214712 ) ) ;
#3505=CYLINDRICAL_SURFACE ( 'NONE', #10583, 30.16249999999999432 ) ;
#3509=CARTESIAN_POINT ( 'NONE',  ( 48.78323016782857735, 37.11476346399999926, -25.79158832643865651 ) ) ;
#3522=DIRECTION ( 'NONE',  ( -0.6702301885068652210, 0.000000000000000000, -0.7421532822901560911 ) ) ;
#3524=VERTEX_POINT ( 'NONE', #12887 ) ;
#3525=CARTESIAN_POINT ( 'NONE',  ( 49.15122309515935228, 0.000000000000000000, -25.07506492104907991 ) ) ;
#3526=SHAPE_REPRESENTATION ( 'Split Webbing Winding Axle', ( #2234 ), #5057 ) ;
#3529=AXIS2_PLACEMENT_3D ( 'NONE', #12859, #4446, #5157 ) ;
#3531=DIRECTION ( 'NONE',  ( 0.000000000000000000, -1.000000000000000000, -0.000000000000000000 ) ) ;
#3535=EDGE_CURVE ( 'NONE', #18152, #4527, #4800, .T. ) ;
#3536=CARTESIAN_POINT ( 'NONE',  ( 32.52436584422698473, 0.000000000000000000, 1.884807767196291284 ) ) ;
#3537=EDGE_CURVE ( 'NONE', #1050, #7386, #1467, .T. ) ;
#3538=ORIENTED_EDGE ( 'NONE', *, *, #18968, .T. ) ;
#3540=DIRECTION ( 'NONE',  ( 0.000000000000000000, -1.000000000000000000, -0.000000000000000000 ) ) ;
#3541=CARTESIAN_POINT ( 'NONE',  ( 50.29383871662588490, 32.54502000000000095, -28.02957329025317179 ) ) ;
#3547=VERTEX_POINT ( 'NONE', #13104 ) ;
#3557=CIRCLE ( 'NONE', #7453, 0.5079999999999996740 ) ;
#3559=EDGE_CURVE ( 'NONE', #1126, #15606, #5100, .T. ) ;
#3565=CARTESIAN_POINT ( 'NONE',  ( 30.25543876212147509, 32.54502000000000095, -19.39939755251907272 ) ) ;
#3575=DIRECTION ( 'NONE',  ( 0.7421532822901579785, 0.000000000000000000, -0.6702301885068628895 ) ) ;
#3578=DIRECTION ( 'NONE',  ( 0.000000000000000000, -1.000000000000000000, -0.000000000000000000 ) ) ;
#3584=CARTESIAN_POINT ( 'NONE',  ( 50.29383871662588490, -1.983739999999999837, -28.02957329025317179 ) ) ;
#3588=AXIS2_PLACEMENT_3D ( 'NONE', #12638, #19470, #21126 ) ;
#3595=CIRCLE ( 'NONE', #21595, 0.7950199999999993938 ) ;
#3598=DIRECTION ( 'NONE',  ( 0.000000000000000000, 1.000000000000000000, -0.000000000000000000 ) ) ;
#3604=AXIS2_PLACEMENT_3D ( 'NONE', #13602, #15378, #3964 ) ;
#3611=AXIS2_PLACEMENT_3D ( 'NONE', #9381, #976, #7726 ) ;
#3619=AXIS2_PLACEMENT_3D ( 'NONE', #9653, #19702, #13319 ) ;
#3625=CIRCLE ( 'NONE', #7165, 0.5080000000000023386 ) ;
#3637=AXIS2_PLACEMENT_3D ( 'NONE', #15254, #6832, #21756 ) ;
#3651=ORIENTED_EDGE ( 'NONE', *, *, #14153, .T. ) ;
#3655=CARTESIAN_POINT ( 'NONE',  ( 53.84486179190094646, 32.54502000000000095, -6.412645463410259872 ) ) ;
#3661=ORIENTED_EDGE ( 'NONE', *, *, #9023, .F. ) ;
#3662=FACE_OUTER_BOUND ( 'NONE', #2631, .T. ) ;
#3667=CYLINDRICAL_SURFACE ( 'NONE', #13017, 0.5080000000000007843 ) ;
#3669=VECTOR ( 'NONE', #3531, 1000.000000000000000 ) ;
#3672=CARTESIAN_POINT ( 'NONE',  ( 38.99879864891609316, 37.69823060749433807, -3.901399344704656436 ) ) ;
#3680=DIRECTION ( 'NONE',  ( 0.000000000000000000, 1.000000000000000000, 0.000000000000000000 ) ) ;
#3685=ADVANCED_FACE ( 'NONE', ( #7967, #12965, #16709 ), #14513, .F. ) ;
#3687=FACE_OUTER_BOUND ( 'NONE', #4070, .T. ) ;
#3691=DIRECTION ( 'NONE',  ( -0.8667647648559581031, 0.000000000000000000, -0.4987171968201974948 ) ) ;
#3693=ORIENTED_EDGE ( 'NONE', *, *, #14369, .T. ) ;
#3701=ORIENTED_EDGE ( 'NONE', *, *, #19264, .T. ) ;
#3709=ORIENTED_EDGE ( 'NONE', *, *, #17974, .T. ) ;
#3713=ORIENTED_EDGE ( 'NONE', *, *, #20042, .F. ) ;
#3719=LINE ( 'NONE', #15347, #6394 ) ;
#3720=ORIENTED_EDGE ( 'NONE', *, *, #14274, .T. ) ;
#3725=EDGE_CURVE ( 'NONE', #19311, #7286, #16807, .T. ) ;
#3730=AXIS2_PLACEMENT_3D ( 'NONE', #17397, #8745, #10527 ) ;
#3733=DIRECTION ( 'NONE',  ( -0.7421532822901579785, 0.000000000000000000, 0.6702301885068630005 ) ) ;
#3736=DIRECTION ( 'NONE',  ( 0.9784543669157820256, 0.000000000000000000, 0.2064631973583577473 ) ) ;
#3737=VERTEX_POINT ( 'NONE', #15389 ) ;
#3740=CYLINDRICAL_SURFACE ( 'NONE', #19491, 9.524999999999998579 ) ;
#3741=EDGE_CURVE ( 'NONE', #9035, #9720, #10496, .T. ) ;
#3750=DIRECTION ( 'NONE',  ( -0.1060008583745199739, 0.000000000000000000, -0.9943660382494290406 ) ) ;
#3753=ORIENTED_EDGE ( 'NONE', *, *, #758, .F. ) ;
#3756=ORIENTED_EDGE ( 'NONE', *, *, #17014, .T. ) ;
#3758=CARTESIAN_POINT ( 'NONE',  ( 52.49113927203449492, -6.356984999999999886, -16.14695822742181619 ) ) ;
#3760=CARTESIAN_POINT ( 'NONE',  ( 54.55586098912687731, -9.531985000000000596, -6.056925149195119040 ) ) ;
#3763=DIRECTION ( 'NONE',  ( 0.1060008583745224581, 0.000000000000000000, 0.9943660382494288186 ) ) ;
#3766=DIRECTION ( 'NONE',  ( 0.000000000000000000, -1.000000000000000000, -0.000000000000000000 ) ) ;
#3767=CARTESIAN_POINT ( 'NONE',  ( 52.36707797519913044, -5.757307957063426684, -17.43673301238325379 ) ) ;
#3770=VERTEX_POINT ( 'NONE', #18890 ) ;
#3775=ORIENTED_EDGE ( 'NONE', *, *, #12412, .T. ) ;
#3784=AXIS2_PLACEMENT_3D ( 'NONE', #11766, #8422, #6990 ) ;
#3788=DIRECTION ( 'NONE',  ( 0.1060008583745200711, 0.000000000000000000, 0.9943660382494290406 ) ) ;
#3790=LINE ( 'NONE', #19147, #17678 ) ;
#3791=CARTESIAN_POINT ( 'NONE',  ( 64.66604708500285881, 0.000000000000000000, -11.54913207920052720 ) ) ;
#3793=DIRECTION ( 'NONE',  ( 0.000000000000000000, -1.000000000000000000, -0.000000000000000000 ) ) ;
#3794=EDGE_CURVE ( 'NONE', #1425, #10463, #20099, .T. ) ;
#3795=CARTESIAN_POINT ( 'NONE',  ( 32.42378190387104553, 32.54502000000000095, -18.15178106273469183 ) ) ;
#3797=CARTESIAN_POINT ( 'NONE',  ( 30.41963056417667488, 34.52875999999999834, -8.653862521447852174 ) ) ;
#3814=CARTESIAN_POINT ( 'NONE',  ( 53.10651001381376091, -7.547610000000002373, -16.70269254552787075 ) ) ;
#3817=ADVANCED_FACE ( 'NONE', ( #20314 ), #10060, .T. ) ;
#3822=CARTESIAN_POINT ( 'NONE',  ( 53.08681243024872742, 40.07829845791615497, -16.72443647849243575 ) ) ;
#3823=ORIENTED_EDGE ( 'NONE', *, *, #13613, .T. ) ;
#3828=CARTESIAN_POINT ( 'NONE',  ( 64.19677489640052670, -1.983739999999999837, -11.74367670905533423 ) ) ;
#3834=CARTESIAN_POINT ( 'NONE',  ( 38.96848998618624904, 40.07865999999999929, -3.934807454472129429 ) ) ;
#3837=DIRECTION ( 'NONE',  ( -0.9724402360367336851, 0.000000000000000000, 0.2331522835762537549 ) ) ;
#3844=VECTOR ( 'NONE', #13436, 1000.000000000000000 ) ;
#3848=CARTESIAN_POINT ( 'NONE',  ( 61.04701390398659555, 34.52875999999999834, -15.15157976445104993 ) ) ;
#3851=ORIENTED_EDGE ( 'NONE', *, *, #1681, .F. ) ;
#3855=CARTESIAN_POINT ( 'NONE',  ( 48.58367710892853353, -1.983739999999999837, -25.32442392637788231 ) ) ;
#3856=VERTEX_POINT ( 'NONE', #21774 ) ;
#3862=ORIENTED_EDGE ( 'NONE', *, *, #5153, .T. ) ;
#3871=CARTESIAN_POINT ( 'NONE',  ( 38.46727988002800913, -7.323121355281222655, -4.536819773745172313 ) ) ;
#3872=CARTESIAN_POINT ( 'NONE',  ( 31.68988926855799448, 0.000000000000000000, 1.626235259850384418 ) ) ;
#3880=EDGE_LOOP ( 'NONE', ( #9597, #11365, #14261, #1942 ) ) ;
#3890=FACE_OUTER_BOUND ( 'NONE', #4134, .T. ) ;
#3891=AXIS2_PLACEMENT_3D ( 'NONE', #3142, #16748, #1263 ) ;
#3899=DIRECTION ( 'NONE',  ( -0.9987059298363656357, 0.000000000000000000, -0.05085730733808393328 ) ) ;
#3902=CARTESIAN_POINT ( 'NONE',  ( 39.27728671717661513, 0.000000000000000000, -23.95520057284206672 ) ) ;
#3908=VERTEX_POINT ( 'NONE', #5745 ) ;
#3909=LINE ( 'NONE', #17613, #13850 ) ;
#3918=CIRCLE ( 'NONE', #6733, 0.5080000000000034488 ) ;
#3919=EDGE_CURVE ( 'NONE', #20253, #7504, #18523, .T. ) ;
#3926=CARTESIAN_POINT ( 'NONE',  ( 56.91751438644678984, 34.52875999999999834, -20.96198986413465448 ) ) ;
#3931=ORIENTED_EDGE ( 'NONE', *, *, #9789, .F. ) ;
#3939=CARTESIAN_POINT ( 'NONE',  ( 50.52547294529469468, 38.88803500000000213, -18.64987929725020521 ) ) ;
#3943=VECTOR ( 'NONE', #19960, 1000.000000000000000 ) ;
#3947=CIRCLE ( 'NONE', #1471, 30.16249999999998721 ) ;
#3949=ORIENTED_EDGE ( 'NONE', *, *, #4679, .F. ) ;
#3953=CIRCLE ( 'NONE', #11369, 0.7950199999999985057 ) ;
#3956=CARTESIAN_POINT ( 'NONE',  ( 59.90456643211351917, 2.586003464000000029, -2.926035437812116946 ) ) ;
#3957=CARTESIAN_POINT ( 'NONE',  ( 30.50878709810603340, 29.95901653600000003, -19.83971405306587954 ) ) ;
#3962=B_SPLINE_CURVE_WITH_KNOTS ( 'NONE', 3,
 ( #17142, #5408, #1984, #12173, #10169, #18670, #3767, #11732, #10504, #16913, #7715, #13621, #17249, #18467, #3335, #1653, #8394, #15285 ),
 .UNSPECIFIED., .F., .F.,
 ( 4, 2, 2, 2, 2, 2, 2, 2, 4 ),
 ( 0.003754349818373628987, 0.004223755935673022613, 0.004693162052972417106, 0.005162568170271811599, 0.005631974287571205225, 0.006101380404870598850, 0.006570786522169993343, 0.007040192639469387836, 0.007509598756768781462 ),
 .UNSPECIFIED. ) ;
#3964=DIRECTION ( 'NONE',  ( 0.000000000000000000, -1.000000000000000000, -0.000000000000000000 ) ) ;
#3969=VERTEX_POINT ( 'NONE', #3872 ) ;
#3970=ORIENTED_EDGE ( 'NONE', *, *, #12995, .F. ) ;
#3974=VERTEX_POINT ( 'NONE', #10724 ) ;
#3975=EDGE_CURVE ( 'NONE', #2248, #2705, #1232, .T. ) ;
#3977=CIRCLE ( 'NONE', #16346, 0.5080000000000012284 ) ;
#3978=CARTESIAN_POINT ( 'NONE',  ( 59.89111109153450485, 34.52875999999999834, -22.14529389979288965 ) ) ;
#3980=LINE ( 'NONE', #3760, #7221 ) ;
#3988=VECTOR ( 'NONE', #11861, 1000.000000000000000 ) ;
#3989=ORIENTED_EDGE ( 'NONE', *, *, #15440, .F. ) ;
#4003=ADVANCED_FACE ( 'NONE', ( #2085 ), #2644, .T. ) ;
#4004=DIRECTION ( 'NONE',  ( 0.7421532822901572013, 0.000000000000000000, -0.6702301885068637777 ) ) ;
#4011=DIRECTION ( 'NONE',  ( 0.7421532822901579785, 0.000000000000000000, -0.6702301885068628895 ) ) ;
#4014=DIRECTION ( 'NONE',  ( 0.7421532822901569793, 0.000000000000000000, -0.6702301885068642218 ) ) ;
#4016=DIRECTION ( 'NONE',  ( -0.07875956036501312318, 0.000000000000000000, 0.9968936410927243807 ) ) ;
#4027=ORIENTED_EDGE ( 'NONE', *, *, #15919, .T. ) ;
#4030=AXIS2_PLACEMENT_3D ( 'NONE', #14713, #8908, #2279 ) ;
#4033=VECTOR ( 'NONE', #2083, 1000.000000000000114 ) ;
#4035=CARTESIAN_POINT ( 'NONE',  ( 30.47347900023190803, 0.000000000000000000, -8.148724574017967015 ) ) ;
#4049=CARTESIAN_POINT ( 'NONE',  ( 43.49132289107146931, 0.000000000000000000, 4.686923926377883021 ) ) ;
#4054=CARTESIAN_POINT ( 'NONE',  ( 39.82201269448036385, -6.200394330680151889, -3.101178208336223818 ) ) ;
#4055=ORIENTED_EDGE ( 'NONE', *, *, #20746, .F. ) ;
#4059=ORIENTED_EDGE ( 'NONE', *, *, #12490, .T. ) ;
#4060=DIRECTION ( 'NONE',  ( 0.9129422336036127072, 0.000000000000000000, -0.4080888115384278536 ) ) ;
#4064=AXIS2_PLACEMENT_3D ( 'NONE', #2535, #2202, #8943 ) ;
#4065=FACE_OUTER_BOUND ( 'NONE', #18135, .T. ) ;
#4068=DIRECTION ( 'NONE',  ( 0.3928209820863007851, 0.000000000000000000, -0.9196149607486571176 ) ) ;
#4070=EDGE_LOOP ( 'NONE', ( #8707, #20950, #17413, #12279 ) ) ;
#4072=EDGE_CURVE ( 'NONE', #8133, #17060, #11118, .T. ) ;
#4074=CARTESIAN_POINT ( 'NONE',  ( 46.03750000000000142, -9.531985000000000596, -10.31874999999999964 ) ) ;
#4078=VERTEX_POINT ( 'NONE', #21314 ) ;
#4089=CARTESIAN_POINT ( 'NONE',  ( 27.87822510359947614, 0.000000000000000000, -8.893823290944665061 ) ) ;
#4094=ORIENTED_EDGE ( 'NONE', *, *, #20018, .T. ) ;
#4098=CARTESIAN_POINT ( 'NONE',  ( 30.50878709810603340, -1.983739999999999837, -19.83971405306587954 ) ) ;
#4099=DIRECTION ( 'NONE',  ( 0.000000000000000000, 1.000000000000000000, -0.000000000000000000 ) ) ;
#4102=ORIENTED_EDGE ( 'NONE', *, *, #5574, .T. ) ;
#4108=CARTESIAN_POINT ( 'NONE',  ( 38.97454265763864356, 37.69740999999999786, -3.928105264594607071 ) ) ;
#4111=EDGE_CURVE ( 'NONE', #97, #14616, #14714, .T. ) ;
#4134=EDGE_LOOP ( 'NONE', ( #20667, #11265, #16524, #15462 ) ) ;
#4139=ADVANCED_FACE ( 'NONE', ( #6510 ), #13270, .T. ) ;
#4140=DIRECTION ( 'NONE',  ( 0.000000000000000000, 1.000000000000000000, -0.000000000000000000 ) ) ;
#4142=DIRECTION ( 'NONE',  ( 0.000000000000000000, 1.000000000000000000, 0.000000000000000000 ) ) ;
#4145=DIRECTION ( 'NONE',  ( 0.000000000000000000, 1.000000000000000000, 0.000000000000000000 ) ) ;
#4149=CARTESIAN_POINT ( 'NONE',  ( 52.65752393886089067, 39.94029975385505082, -17.16880761802969957 ) ) ;
#4156=EDGE_LOOP ( 'NONE', ( #17793, #20594, #95, #8512 ) ) ;
#4158=CARTESIAN_POINT ( 'NONE',  ( 39.70799623749501706, -5.757505969760286391, -3.200701455436412601 ) ) ;
#4159=ORIENTED_EDGE ( 'NONE', *, *, #11354, .T. ) ;
#4163=VERTEX_POINT ( 'NONE', #14817 ) ;
#4164=DIRECTION ( 'NONE',  ( -0.9987059298363656357, 0.000000000000000000, -0.05085730733808393328 ) ) ;
#4165=EDGE_CURVE ( 'NONE', #2030, #13169, #14691, .T. ) ;
#4169=ORIENTED_EDGE ( 'NONE', *, *, #2312, .T. ) ;
#4171=DIRECTION ( 'NONE',  ( -0.000000000000000000, -1.000000000000000000, 0.000000000000000000 ) ) ;
#4172=CARTESIAN_POINT ( 'NONE',  ( 38.28489021960990613, 38.88803500000000213, 2.732679409805250703 ) ) ;
#4173=VERTEX_POINT ( 'NONE', #16470 ) ;
#4175=FACE_OUTER_BOUND ( 'NONE', #9255, .T. ) ;
#4178=ORIENTED_EDGE ( 'NONE', *, *, #18406, .T. ) ;
#4187=B_SPLINE_CURVE_WITH_KNOTS ( 'NONE', 3,
 ( #21557, #19462, #9509, #4765 ),
 .UNSPECIFIED., .F., .F.,
 ( 4, 4 ),
 ( 0.008316203670685974950, 0.009146310752383313147 ),
 .UNSPECIFIED. ) ;
#4189=CARTESIAN_POINT ( 'NONE',  ( 64.66604708500285881, -1.983739999999999837, -11.54913207920052720 ) ) ;
#4191=DIRECTION ( 'NONE',  ( 0.000000000000000000, 1.000000000000000000, 0.000000000000000000 ) ) ;
#4193=VERTEX_POINT ( 'NONE', #4420 ) ;
#4195=CARTESIAN_POINT ( 'NONE',  ( 31.02798609601340729, 34.52875999999999834, -5.485920235548950252 ) ) ;
#4204=PLANE ( 'NONE',  #7124 ) ;
#4209=VECTOR ( 'NONE', #18646, 1000.000000000000000 ) ;
#4223=AXIS2_PLACEMENT_3D ( 'NONE', #19177, #7464, #16104 ) ;
#4224=CARTESIAN_POINT ( 'NONE',  ( 39.00487391864218267, 37.69864044684034354, -3.894748490052650780 ) ) ;
#4226=DIRECTION ( 'NONE',  ( -0.7532174416907914116, 0.000000000000000000, -0.6577716059034314222 ) ) ;
#4230=CARTESIAN_POINT ( 'NONE',  ( 61.04701390398659555, 0.000000000000000000, -15.15157976445104993 ) ) ;
#4231=VECTOR ( 'NONE', #14776, 1000.000000000000000 ) ;
#4248=AXIS2_PLACEMENT_3D ( 'NONE', #16881, #20186, #406 ) ;
#4249=VECTOR ( 'NONE', #3598, 1000.000000000000000 ) ;
#4253=CARTESIAN_POINT ( 'NONE',  ( 39.93069333241964358, 39.05073723955329967, -3.008993689095917023 ) ) ;
#4255=CARTESIAN_POINT ( 'NONE',  ( 61.60152099976809126, 32.54502000000000095, -12.48877542598203405 ) ) ;
#4258=CARTESIAN_POINT ( 'NONE',  ( 52.19854938732527216, 38.88803500000000213, -17.58284632693144189 ) ) ;
#4263=AXIS2_PLACEMENT_3D ( 'NONE', #11759, #1675, #10089 ) ;
#4265=DIRECTION ( 'NONE',  ( 0.9943660382494290406, 0.000000000000000000, -0.1060008583745199739 ) ) ;
#4268=EDGE_CURVE ( 'NONE', #4911, #8326, #16091, .T. ) ;
#4270=CARTESIAN_POINT ( 'NONE',  ( 30.24348838687780727, 34.52875999999999834, -20.27293523655082552 ) ) ;
#4273=ORIENTED_EDGE ( 'NONE', *, *, #1727, .T. ) ;
#4278=ORIENTED_EDGE ( 'NONE', *, *, #20989, .T. ) ;
#4280=AXIS2_PLACEMENT_3D ( 'NONE', #4074, #4407, #11033 ) ;
#4287=AXIS2_PLACEMENT_3D ( 'NONE', #7337, #2016, #15538 ) ;
#4293=CARTESIAN_POINT ( 'NONE',  ( 37.07154142533928365, -6.356984999999999886, -2.340318470350700508 ) ) ;
#4294=VERTEX_POINT ( 'NONE', #293 ) ;
#4296=EDGE_CURVE ( 'NONE', #11391, #17636, #10137, .T. ) ;
#4300=CIRCLE ( 'NONE', #16653, 1.190625000000000488 ) ;
#4302=AXIS2_PLACEMENT_3D ( 'NONE', #15532, #8867, #15862 ) ;
#4303=CIRCLE ( 'NONE', #18755, 0.5080000000000034488 ) ;
#4309=EDGE_LOOP ( 'NONE', ( #3331, #3538, #20402, #3851 ) ) ;
#4311=DIRECTION ( 'NONE',  ( 0.000000000000000000, -1.000000000000000000, -0.000000000000000000 ) ) ;
#4323=EDGE_CURVE ( 'NONE', #18042, #7386, #16783, .T. ) ;
#4324=FACE_OUTER_BOUND ( 'NONE', #7605, .T. ) ;
#4330=CIRCLE ( 'NONE', #19138, 30.16249999999998721 ) ;
#4333=CIRCLE ( 'NONE', #12454, 0.5079999999999965654 ) ;
#4340=CARTESIAN_POINT ( 'NONE',  ( 34.38097451710952868, 34.52875999999999834, 0.2081255904771098786 ) ) ;
#4341=CARTESIAN_POINT ( 'NONE',  ( 59.65121809612895731, 32.54502000000000095, -2.485718937265306572 ) ) ;
#4344=DIRECTION ( 'NONE',  ( 0.000000000000000000, -1.000000000000000000, -0.000000000000000000 ) ) ;
#4345=AXIS2_PLACEMENT_3D ( 'NONE', #5326, #6661, #2008 ) ;
#4352=FACE_BOUND ( 'NONE', #13992, .T. ) ;
#4355=VECTOR ( 'NONE', #12247, 1000.000000000000000 ) ;
#4357=CARTESIAN_POINT ( 'NONE',  ( 59.65121809612895731, 34.52875999999999834, -2.485718937265306572 ) ) ;
#4359=AXIS2_PLACEMENT_3D ( 'NONE', #1144, #11206, #14870 ) ;
#4362=CARTESIAN_POINT ( 'NONE',  ( 53.92979111630304345, -6.519632010286108503, -15.65141968183250754 ) ) ;
#4363=DIRECTION ( 'NONE',  ( 0.3928209820863022839, 0.000000000000000000, -0.9196149607486564515 ) ) ;
#4364=EDGE_CURVE ( 'NONE', #8109, #13937, #15470, .T. ) ;
#4370=CARTESIAN_POINT ( 'NONE',  ( 47.80475250345343596, 38.88803500000000213, -11.91473563638196786 ) ) ;
#4371=ORIENTED_EDGE ( 'NONE', *, *, #17597, .F. ) ;
#4379=EDGE_CURVE ( 'NONE', #20373, #9905, #1949, .T. ) ;
#4385=CARTESIAN_POINT ( 'NONE',  ( 42.66304184606194383, 0.000000000000000000, -19.22597499813143784 ) ) ;
#4388=VECTOR ( 'NONE', #7512, 1000.000000000000000 ) ;
#4390=ORIENTED_EDGE ( 'NONE', *, *, #18333, .T. ) ;
#4392=CARTESIAN_POINT ( 'NONE',  ( 52.79771328282338771, 34.52875999999999834, 3.317700572842066986 ) ) ;
#4396=DIRECTION ( 'NONE',  ( 0.07875956036501312318, 0.000000000000000000, -0.9968936410927243807 ) ) ;
#4402=VECTOR ( 'NONE', #9805, 1000.000000000000114 ) ;
#4403=ORIENTED_EDGE ( 'NONE', *, *, #14971, .F. ) ;
#4405=EDGE_CURVE ( 'NONE', #18389, #12286, #7678, .T. ) ;
#4407=DIRECTION ( 'NONE',  ( 0.000000000000000000, 1.000000000000000000, 0.000000000000000000 ) ) ;
#4410=ORIENTED_EDGE ( 'NONE', *, *, #19358, .F. ) ;
#4411=ORIENTED_EDGE ( 'NONE', *, *, #19101, .F. ) ;
#4414=ORIENTED_EDGE ( 'NONE', *, *, #14225, .T. ) ;
#4418=CARTESIAN_POINT ( 'NONE',  ( 49.72033008250774344, 32.54502000000000095, -2.687827786179598277 ) ) ;
#4420=CARTESIAN_POINT ( 'NONE',  ( 41.45112526417833010, 0.000000000000000000, 7.778260066349530710 ) ) ;
#4423=ADVANCED_FACE ( 'NONE', ( #1732 ), #8472, .T. ) ;
#4426=DIRECTION ( 'NONE',  ( 0.000000000000000000, -1.000000000000000000, -0.000000000000000000 ) ) ;
#4430=VERTEX_POINT ( 'NONE', #10580 ) ;
#4435=ORIENTED_EDGE ( 'NONE', *, *, #21131, .T. ) ;
#4446=DIRECTION ( 'NONE',  ( -0.000000000000000000, -1.000000000000000000, 0.000000000000000000 ) ) ;
#4449=EDGE_CURVE ( 'NONE', #16972, #2587, #18537, .T. ) ;
#4452=CARTESIAN_POINT ( 'NONE',  ( 52.91086381164393515, -1.983739999999999837, 3.812938856729753301 ) ) ;
#4456=DIRECTION ( 'NONE',  ( 0.000000000000000000, 1.000000000000000000, 0.000000000000000000 ) ) ;
#4463=VERTEX_POINT ( 'NONE', #5486 ) ;
#4464=CARTESIAN_POINT ( 'NONE',  ( 31.68988926855799448, 32.54502000000000095, 1.626235259850384418 ) ) ;
#4466=ORIENTED_EDGE ( 'NONE', *, *, #5218, .F. ) ;
#4467=DIRECTION ( 'NONE',  ( 0.000000000000000000, 1.000000000000000000, 0.000000000000000000 ) ) ;
#4471=EDGE_CURVE ( 'NONE', #18470, #968, #21363, .T. ) ;
#4472=DIRECTION ( 'NONE',  ( 0.1060008583745224581, 0.000000000000000000, 0.9943660382494288186 ) ) ;
#4475=ORIENTED_EDGE ( 'NONE', *, *, #8715, .F. ) ;
#4477=CARTESIAN_POINT ( 'NONE',  ( 47.80475250345343596, -6.356985000000002550, -11.91473563638196786 ) ) ;
#4480=AXIS2_PLACEMENT_3D ( 'NONE', #6338, #11323, #14671 ) ;
#4483=CARTESIAN_POINT ( 'NONE',  ( 59.52193197173441774, 0.000000000000000000, -3.260183413611184911 ) ) ;
#4495=VECTOR ( 'NONE', #14829, 1000.000000000000000 ) ;
#4499=CARTESIAN_POINT ( 'NONE',  ( 42.94469661997857912, -76.79125307200000350, -18.48251861828712705 ) ) ;
#4501=ORIENTED_EDGE ( 'NONE', *, *, #1116, .F. ) ;
#4502=ORIENTED_EDGE ( 'NONE', *, *, #17880, .T. ) ;
#4516=CARTESIAN_POINT ( 'NONE',  ( 39.22866504299416590, 37.71595759399457393, -3.656247628902255631 ) ) ;
#4523=CARTESIAN_POINT ( 'NONE',  ( 53.84486179190094646, -9.531985000000000596, -6.412645463410259872 ) ) ;
#4526=ORIENTED_EDGE ( 'NONE', *, *, #1137, .T. ) ;
#4527=VERTEX_POINT ( 'NONE', #7162 ) ;
#4534=DIRECTION ( 'NONE',  ( 0.05085730733808393328, 0.000000000000000000, -0.9987059298363656357 ) ) ;
#4544=DIRECTION ( 'NONE',  ( -0.6702301885068628895, 0.000000000000000000, -0.7421532822901579785 ) ) ;
#4546=PLANE ( 'NONE',  #20369 ) ;
#4557=ORIENTED_EDGE ( 'NONE', *, *, #9167, .T. ) ;
#4563=ADVANCED_FACE ( 'NONE', ( #2172 ), #5377, .T. ) ;
#4566=EDGE_CURVE ( 'NONE', #7945, #16183, #10419, .T. ) ;
#4568=ORIENTED_EDGE ( 'NONE', *, *, #15488, .F. ) ;
#4569=AXIS2_PLACEMENT_3D ( 'NONE', #20852, #12585, #4171 ) ;
#4572=CARTESIAN_POINT ( 'NONE',  ( 38.55125416157952856, -5.304186826770175500, -4.427761586073884814 ) ) ;
#4575=FACE_OUTER_BOUND ( 'NONE', #2758, .T. ) ;
#4582=DIRECTION ( 'NONE',  ( -0.9784543669157824697, 0.000000000000000000, -0.2064631973583561375 ) ) ;
#4588=CYLINDRICAL_SURFACE ( 'NONE', #8158, 0.5080000000000006732 ) ;
#4590=( NAMED_UNIT ( * ) PLANE_ANGLE_UNIT ( ) SI_UNIT ( $, .RADIAN. ) );
#4592=ADVANCED_FACE ( 'NONE', ( #7271 ), #14032, .T. ) ;
#4606=AXIS2_PLACEMENT_3D ( 'NONE', #15525, #683, #4226 ) ;
#4607=DIRECTION ( 'NONE',  ( 0.000000000000000000, 1.000000000000000000, -0.000000000000000000 ) ) ;
#4616=ORIENTED_EDGE ( 'NONE', *, *, #4268, .F. ) ;
#4622=VECTOR ( 'NONE', #17750, 1000.000000000000000 ) ;
#4624=DIRECTION ( 'NONE',  ( -0.5222415575336509797, 0.000000000000000000, -0.8527976052879290281 ) ) ;
#4625=CARTESIAN_POINT ( 'NONE',  ( 39.39227298748875228, 37.79827878291772691, -3.494347496384869523 ) ) ;
#4629=AXIS2_PLACEMENT_3D ( 'NONE', #3525, #16010, #5912 ) ;
#4635=CARTESIAN_POINT ( 'NONE',  ( 59.89111109153450485, 32.54502000000000095, -22.14529389979288965 ) ) ;
#4636=EDGE_CURVE ( 'NONE', #17408, #12286, #16909, .T. ) ;
#4637=CARTESIAN_POINT ( 'NONE',  ( 53.70914399163670083, 39.62082658259355838, -15.96531164363307376 ) ) ;
#4638=ORIENTED_EDGE ( 'NONE', *, *, #7748, .F. ) ;
#4643=ORIENTED_EDGE ( 'NONE', *, *, #3304, .F. ) ;
#4646=EDGE_CURVE ( 'NONE', #15022, #6484, #2673, .T. ) ;
#4647=EDGE_CURVE ( 'NONE', #3173, #17565, #10082, .T. ) ;
#4648=ADVANCED_FACE ( 'NONE', ( #11760 ), #3033, .T. ) ;
#4651=AXIS2_PLACEMENT_3D ( 'NONE', #9516, #8075, #16286 ) ;
#4659=ORIENTED_EDGE ( 'NONE', *, *, #12053, .T. ) ;
#4665=DIRECTION ( 'NONE',  ( -0.4080888115384288528, 0.000000000000000000, -0.9129422336036122632 ) ) ;
#4668=LINE ( 'NONE', #1011, #7119 ) ;
#4676=AXIS2_PLACEMENT_3D ( 'NONE', #3655, #6745, #16716 ) ;
#4679=EDGE_CURVE ( 'NONE', #1990, #20092, #13998, .T. ) ;
#4689=CARTESIAN_POINT ( 'NONE',  ( 32.55306802826559220, 0.000000000000000000, -17.37731658638881527 ) ) ;
#4696=ORIENTED_EDGE ( 'NONE', *, *, #10338, .F. ) ;
#4700=VECTOR ( 'NONE', #8270, 1000.000000000000000 ) ;
#4701=ORIENTED_EDGE ( 'NONE', *, *, #19356, .F. ) ;
#4709=DIRECTION ( 'NONE',  ( 0.000000000000000000, 1.000000000000000000, 0.000000000000000000 ) ) ;
#4711=ORIENTED_EDGE ( 'NONE', *, *, #14121, .F. ) ;
#4712=VECTOR ( 'NONE', #1028, 1000.000000000000000 ) ;
#4715=ORIENTED_EDGE ( 'NONE', *, *, #2919, .F. ) ;
#4725=CARTESIAN_POINT ( 'NONE',  ( 44.27024749654656688, -6.356984999999999886, -8.722764363618033201 ) ) ;
#4728=ORIENTED_EDGE ( 'NONE', *, *, #21525, .T. ) ;
#4741=DIRECTION ( 'NONE',  ( -0.7421532822901579785, 0.000000000000000000, 0.6702301885068630005 ) ) ;
#4747=EDGE_CURVE ( 'NONE', #10568, #19175, #14989, .T. ) ;
#4754=EDGE_LOOP ( 'NONE', ( #6546, #13349, #13456, #21184 ) ) ;
#4756=DIRECTION ( 'NONE',  ( 0.6702301885068632226, 0.000000000000000000, 0.7421532822901576454 ) ) ;
#4757=AXIS2_PLACEMENT_3D ( 'NONE', #7560, #21043, #10982 ) ;
#4765=CARTESIAN_POINT ( 'NONE',  ( 52.49113927203492125, -7.547609999999999708, -16.14695822742135078 ) ) ;
#4777=AXIS2_PLACEMENT_3D ( 'NONE', #7674, #2807, #4363 ) ;
#4791=DIRECTION ( 'NONE',  ( -0.9784543669157944601, 0.000000000000000000, -0.2064631973582987945 ) ) ;
#4799=LINE ( 'NONE', #18178, #21271 ) ;
#4800=LINE ( 'NONE', #11531, #2276 ) ;
#4806=DIRECTION ( 'NONE',  ( -0.7421532822901579785, 0.000000000000000000, 0.6702301885068630005 ) ) ;
#4814=DIRECTION ( 'NONE',  ( 0.6702301885068630005, 0.000000000000000000, 0.7421532822901579785 ) ) ;
#4828=DIRECTION ( 'NONE',  ( 0.000000000000000000, 1.000000000000000000, 0.000000000000000000 ) ) ;
#4829=ORIENTED_EDGE ( 'NONE', *, *, #17099, .F. ) ;
#4837=CARTESIAN_POINT ( 'NONE',  ( 52.94929985906785674, 37.69729076100792753, -16.57396907547657605 ) ) ;
#4840=ORIENTED_EDGE ( 'NONE', *, *, #8550, .F. ) ;
#4851=DIRECTION ( 'NONE',  ( 0.7421532822901569793, 0.000000000000000000, -0.6702301885068642218 ) ) ;
#4854=CARTESIAN_POINT ( 'NONE',  ( 41.71184157647478230, 38.88803500000000213, -2.134205101306931862 ) ) ;
#4863=ORIENTED_EDGE ( 'NONE', *, *, #6811, .F. ) ;
#4872=DIRECTION ( 'NONE',  ( -0.9959941601142525691, 0.000000000000000000, -0.08941830359777946935 ) ) ;
#4882=DIRECTION ( 'NONE',  ( 0.9784543669157820256, 0.000000000000000000, 0.2064631973583577473 ) ) ;
#4883=CYLINDRICAL_SURFACE ( 'NONE', #5652, 1.190625000000000711 ) ;
#4888=CARTESIAN_POINT ( 'NONE',  ( 53.95242430215955665, 38.88803500000000213, -23.51676380836238067 ) ) ;
#4896=ORIENTED_EDGE ( 'NONE', *, *, #15769, .F. ) ;
#4897=DIRECTION ( 'NONE',  ( 0.000000000000000000, 1.000000000000000000, 0.000000000000000000 ) ) ;
#4905=DIRECTION ( 'NONE',  ( 0.000000000000000000, -1.000000000000000000, -0.000000000000000000 ) ) ;
#4910=AXIS2_PLACEMENT_3D ( 'NONE', #302, #15700, #15476 ) ;
#4911=VERTEX_POINT ( 'NONE', #3791 ) ;
#4926=ADVANCED_FACE ( 'NONE', ( #1787 ), #2120, .T. ) ;
#4928=VERTEX_POINT ( 'NONE', #15526 ) ;
#4943=CARTESIAN_POINT ( 'NONE',  ( 37.29356535768673098, -6.356984999999999886, -6.700294045292300105 ) ) ;
#4948=DIRECTION ( 'NONE',  ( 0.7532174416907910786, 0.000000000000000000, 0.6577716059034319773 ) ) ;
#4951=CARTESIAN_POINT ( 'NONE',  ( 53.83113913812347562, 39.20076143050763307, -15.79492098357274443 ) ) ;
#4953=EDGE_CURVE ( 'NONE', #13623, #21520, #8312, .T. ) ;
#4954=ORIENTED_EDGE ( 'NONE', *, *, #872, .T. ) ;
#4959=EDGE_LOOP ( 'NONE', ( #3713, #12711, #1289, #8359 ) ) ;
#4964=CARTESIAN_POINT ( 'NONE',  ( 61.65536943582333151, 34.52875999999999834, -11.98363747855214712 ) ) ;
#4967=CARTESIAN_POINT ( 'NONE',  ( 48.60274532164483929, 38.88803500000000213, -11.03110938465478164 ) ) ;
#4972=EDGE_LOOP ( 'NONE', ( #6075, #12692, #4643, #4159 ) ) ;
#4974=CARTESIAN_POINT ( 'NONE',  ( 31.02798609601340729, 32.54502000000000095, -5.485920235548950252 ) ) ;
#4975=DIRECTION ( 'NONE',  ( 0.6702301885068632226, 0.000000000000000000, 0.7421532822901576454 ) ) ;
#4976=DIRECTION ( 'NONE',  ( 0.000000000000000000, -1.000000000000000000, -0.000000000000000000 ) ) ;
#4991=AXIS2_PLACEMENT_3D ( 'NONE', #13959, #3766, #7072 ) ;
#4993=VECTOR ( 'NONE', #13085, 1000.000000000000114 ) ;
#5003=CYLINDRICAL_SURFACE ( 'NONE', #4263, 30.16250000000000142 ) ;
#5007=EDGE_CURVE ( 'NONE', #2509, #15569, #11146, .T. ) ;
#5009=ORIENTED_EDGE ( 'NONE', *, *, #5352, .F. ) ;
#5012=DIRECTION ( 'NONE',  ( 0.000000000000000000, -1.000000000000000000, -0.000000000000000000 ) ) ;
#5018=DIRECTION ( 'NONE',  ( 0.000000000000000000, 1.000000000000000000, 0.000000000000000000 ) ) ;
#5021=FACE_OUTER_BOUND ( 'NONE', #21760, .T. ) ;
#5025=ORIENTED_EDGE ( 'NONE', *, *, #16213, .T. ) ;
#5026=CIRCLE ( 'NONE', #13182, 0.5080000000000022276 ) ;
#5030=DIRECTION ( 'NONE',  ( 0.000000000000000000, -1.000000000000000000, -0.000000000000000000 ) ) ;
#5032=VECTOR ( 'NONE', #18373, 1000.000000000000000 ) ;
#5040=ORIENTED_EDGE ( 'NONE', *, *, #4566, .F. ) ;
#5050=EDGE_LOOP ( 'NONE', ( #16753, #17727, #16544, #13146 ) ) ;
#5052=AXIS2_PLACEMENT_3D ( 'NONE', #12946, #10249, #4851 ) ;
#5053=LINE ( 'NONE', #10237, #20589 ) ;
#5054=ORIENTED_EDGE ( 'NONE', *, *, #9724, .F. ) ;
#5055=EDGE_CURVE ( 'NONE', #17518, #12957, #20893, .T. ) ;
#5057=( GEOMETRIC_REPRESENTATION_CONTEXT ( 3 ) GLOBAL_UNCERTAINTY_ASSIGNED_CONTEXT ( ( #1926 ) ) GLOBAL_UNIT_ASSIGNED_CONTEXT ( ( #12674, #4590, #6136 ) ) REPRESENTATION_CONTEXT ( 'NONE', 'WORKASPACE' ) );
#5062=EDGE_LOOP ( 'NONE', ( #79, #10861, #17128, #1742 ) ) ;
#5065=DIRECTION ( 'NONE',  ( 0.000000000000000000, 1.000000000000000000, 0.000000000000000000 ) ) ;
#5071=ORIENTED_EDGE ( 'NONE', *, *, #1681, .T. ) ;
#5075=CARTESIAN_POINT ( 'NONE',  ( 39.58386072796550081, 38.88803500000000213, -4.490541772578183100 ) ) ;
#5084=EDGE_CURVE ( 'NONE', #17030, #7588, #2174, .T. ) ;
#5096=ORIENTED_EDGE ( 'NONE', *, *, #1116, .T. ) ;
#5100=CIRCLE ( 'NONE', #8265, 0.5079999999999996740 ) ;
#5104=DIRECTION ( 'NONE',  ( 0.000000000000000000, 1.000000000000000000, 0.000000000000000000 ) ) ;
#5105=CARTESIAN_POINT ( 'NONE',  ( 49.28028498622276032, 0.000000000000000000, -25.68670502218146368 ) ) ;
#5108=PLANE ( 'NONE',  #12347 ) ;
#5112=DIRECTION ( 'NONE',  ( 0.000000000000000000, -1.000000000000000000, -0.000000000000000000 ) ) ;
#5118=DIRECTION ( 'NONE',  ( -0.9129422336036514540, 0.000000000000000000, 0.4080888115383414783 ) ) ;
#5126=ORIENTED_EDGE ( 'NONE', *, *, #13613, .F. ) ;
#5129=DIRECTION ( 'NONE',  ( -0.9784543669157950152, 0.000000000000000000, -0.2064631973582961577 ) ) ;
#5136=AXIS2_PLACEMENT_3D ( 'NONE', #9983, #11640, #14873 ) ;
#5142=VERTEX_POINT ( 'NONE', #14522 ) ;
#5143=ORIENTED_EDGE ( 'NONE', *, *, #2925, .T. ) ;
#5153=EDGE_CURVE ( 'NONE', #11670, #8981, #20794, .T. ) ;
#5157=DIRECTION ( 'NONE',  ( 0.7421532822901569793, 0.000000000000000000, -0.6702301885068642218 ) ) ;
#5160=CARTESIAN_POINT ( 'NONE',  ( 46.03750000000000142, -1.983739999999999837, -10.31874999999999964 ) ) ;
#5162=DIRECTION ( 'NONE',  ( -0.7421532822901572013, 0.000000000000000000, 0.6702301885068637777 ) ) ;
#5166=CARTESIAN_POINT ( 'NONE',  ( 50.62387473582167274, -1.983739999999999837, -28.41576006634952734 ) ) ;
#5173=ORIENTED_EDGE ( 'NONE', *, *, #5084, .T. ) ;
#5178=ORIENTED_EDGE ( 'NONE', *, *, #14926, .T. ) ;
#5180=EDGE_CURVE ( 'NONE', #12537, #18019, #3953, .T. ) ;
#5185=FACE_OUTER_BOUND ( 'NONE', #13037, .T. ) ;
#5186=VECTOR ( 'NONE', #16992, 1000.000000000000000 ) ;
#5187=ORIENTED_EDGE ( 'NONE', *, *, #12739, .T. ) ;
#5189=CARTESIAN_POINT ( 'NONE',  ( 48.60274532164400085, -6.356984999999999886, -11.03110938465571245 ) ) ;
#5191=LINE ( 'NONE', #16914, #10313 ) ;
#5192=EDGE_LOOP ( 'NONE', ( #7403, #19658, #6940, #9759 ) ) ;
#5194=LINE ( 'NONE', #12283, #17725 ) ;
#5196=VERTEX_POINT ( 'NONE', #7650 ) ;
#5198=ORIENTED_EDGE ( 'NONE', *, *, #2365, .T. ) ;
#5200=DIRECTION ( 'NONE',  ( 0.000000000000000000, -1.000000000000000000, 0.000000000000000000 ) ) ;
#5201=ADVANCED_FACE ( 'NONE', ( #13396 ), #8189, .T. ) ;
#5212=FACE_OUTER_BOUND ( 'NONE', #12945, .T. ) ;
#5218=EDGE_CURVE ( 'NONE', #3856, #4078, #1807, .T. ) ;
#5224=CARTESIAN_POINT ( 'NONE',  ( 60.38511073144201191, 34.52875999999999834, -22.26373525985038526 ) ) ;
#5229=VERTEX_POINT ( 'NONE', #6307 ) ;
#5234=DIRECTION ( 'NONE',  ( -0.3542738219355860418, 0.000000000000000000, -0.9351417320872557060 ) ) ;
#5241=ORIENTED_EDGE ( 'NONE', *, *, #5502, .T. ) ;
#5242=EDGE_CURVE ( 'NONE', #1819, #18960, #14205, .T. ) ;
#5247=DIRECTION ( 'NONE',  ( 0.000000000000000000, 1.000000000000000000, 0.000000000000000000 ) ) ;
#5251=ORIENTED_EDGE ( 'NONE', *, *, #5180, .F. ) ;
#5273=PLANE ( 'NONE',  #15273 ) ;
#5279=ORIENTED_EDGE ( 'NONE', *, *, #2874, .T. ) ;
#5286=CARTESIAN_POINT ( 'NONE',  ( 49.41195815393805901, 32.54502000000000805, -1.411525001868561224 ) ) ;
#5290=DIRECTION ( 'NONE',  ( 0.000000000000000000, 1.000000000000000000, 0.000000000000000000 ) ) ;
#5292=LINE ( 'NONE', #15502, #13878 ) ;
#5297=ADVANCED_FACE ( 'NONE', ( #1332 ), #17377, .T. ) ;
#5301=EDGE_LOOP ( 'NONE', ( #21409, #15071, #12329, #12333, #18326, #2264 ) ) ;
#5303=DIRECTION ( 'NONE',  ( 0.000000000000000000, 1.000000000000000000, 0.000000000000000000 ) ) ;
#5318=DIRECTION ( 'NONE',  ( -0.05085730733808142834, 0.000000000000000000, 0.9987059298363657467 ) ) ;
#5320=DIRECTION ( 'NONE',  ( 0.000000000000000000, 1.000000000000000000, 0.000000000000000000 ) ) ;
#5321=DIRECTION ( 'NONE',  ( 0.000000000000000000, -1.000000000000000000, -0.000000000000000000 ) ) ;
#5326=CARTESIAN_POINT ( 'NONE',  ( 57.35354854712898742, 2.586003464000000029, -21.22263945788050776 ) ) ;
#5336=CYLINDRICAL_SURFACE ( 'NONE', #4287, 30.16250000000000142 ) ;
#5352=EDGE_CURVE ( 'NONE', #4463, #5142, #15566, .T. ) ;
#5356=ORIENTED_EDGE ( 'NONE', *, *, #18827, .F. ) ;
#5363=CARTESIAN_POINT ( 'NONE',  ( 49.72033008250774344, 42.06303499999999929, -2.687827786179598277 ) ) ;
#5373=AXIS2_PLACEMENT_3D ( 'NONE', #13800, #20736, #10466 ) ;
#5375=CARTESIAN_POINT ( 'NONE',  ( 42.79471501377724252, 32.54502000000000095, 5.049205022181460834 ) ) ;
#5377=CYLINDRICAL_SURFACE ( 'NONE', #15053, 0.5080000000000000071 ) ;
#5380=CARTESIAN_POINT ( 'NONE',  ( 54.88544852023625253, 38.88803500000000213, -18.42785536490203668 ) ) ;
#5384=CARTESIAN_POINT ( 'NONE',  ( 49.79678389823170903, 32.54502000000000095, -28.13445659451038594 ) ) ;
#5388=VERTEX_POINT ( 'NONE', #20423 ) ;
#5392=ORIENTED_EDGE ( 'NONE', *, *, #9775, .T. ) ;
#5402=DIRECTION ( 'NONE',  ( 0.000000000000000000, 1.000000000000000000, 0.000000000000000000 ) ) ;
#5408=CARTESIAN_POINT ( 'NONE',  ( 53.00229660230819917, -5.166360000000002728, -16.81808920586004419 ) ) ;
#5410=ORIENTED_EDGE ( 'NONE', *, *, #19907, .T. ) ;
#5416=ORIENTED_EDGE ( 'NONE', *, *, #8999, .F. ) ;
#5417=CARTESIAN_POINT ( 'NONE',  ( 47.80475250345343596, 38.88803500000000213, -11.91473563638196786 ) ) ;
#5420=DIRECTION ( 'NONE',  ( 0.000000000000000000, -1.000000000000000000, -0.000000000000000000 ) ) ;
#5424=EDGE_CURVE ( 'NONE', #15045, #8192, #20166, .T. ) ;
#5426=ADVANCED_FACE ( 'NONE', ( #15396 ), #221, .T. ) ;
#5438=CARTESIAN_POINT ( 'NONE',  ( 61.02111788801703085, 0.000000000000000000, -5.406220493519755088 ) ) ;
#5447=EDGE_CURVE ( 'NONE', #11597, #3189, #3434, .T. ) ;
#5452=ORIENTED_EDGE ( 'NONE', *, *, #20067, .F. ) ;
#5457=DIRECTION ( 'NONE',  ( 0.9784543669157947932, 0.000000000000000000, 0.2064631973582977953 ) ) ;
#5458=LINE ( 'NONE', #18941, #14299 ) ;
#5481=DIRECTION ( 'NONE',  ( 0.000000000000000000, 1.000000000000000000, 0.000000000000000000 ) ) ;
#5486=CARTESIAN_POINT ( 'NONE',  ( 53.92979111630407374, -6.356984999999459873, -15.65141968182990162 ) ) ;
#5487=DIRECTION ( 'NONE',  ( -0.6702301885068639997, 0.000000000000000000, -0.7421532822901570903 ) ) ;
#5498=ORIENTED_EDGE ( 'NONE', *, *, #3446, .F. ) ;
#5502=EDGE_CURVE ( 'NONE', #7588, #17030, #2899, .T. ) ;
#5503=VERTEX_POINT ( 'NONE', #20545 ) ;
#5510=CARTESIAN_POINT ( 'NONE',  ( 38.23013820809905638, -1.983739999999999837, -14.22485453658974031 ) ) ;
#5522=AXIS2_PLACEMENT_3D ( 'NONE', #11539, #21598, #3137 ) ;
#5531=CARTESIAN_POINT ( 'NONE',  ( 32.42378190387104553, 34.52875999999999834, -18.15178106273469183 ) ) ;
#5545=CYLINDRICAL_SURFACE ( 'NONE', #2879, 0.5080000000000022276 ) ;
#5549=CARTESIAN_POINT ( 'NONE',  ( 61.83151161312219557, 32.54502000000000095, -0.3645647634491749334 ) ) ;
#5550=EDGE_CURVE ( 'NONE', #13568, #16035, #3962, .T. ) ;
#5567=DIRECTION ( 'NONE',  ( -0.4987171968201988270, 0.000000000000000000, 0.8667647648559574369 ) ) ;
#5572=DIRECTION ( 'NONE',  ( -0.6496772031432439531, 0.000000000000000000, 0.7602101891687401691 ) ) ;
#5573=ORIENTED_EDGE ( 'NONE', *, *, #454, .F. ) ;
#5574=EDGE_CURVE ( 'NONE', #14379, #4173, #17393, .T. ) ;
#5576=DIRECTION ( 'NONE',  ( -0.6702301885068628895, 0.000000000000000000, -0.7421532822901579785 ) ) ;
#5580=DIRECTION ( 'NONE',  ( -0.6702301885068632226, 0.000000000000000000, -0.7421532822901577564 ) ) ;
#5581=ORIENTED_EDGE ( 'NONE', *, *, #14126, .T. ) ;
#5594=DIRECTION ( 'NONE',  ( -0.7421532822901572013, 0.000000000000000000, 0.6702301885068637777 ) ) ;
#5599=DIRECTION ( 'NONE',  ( -0.9784543669157947932, 0.000000000000000000, -0.2064631973582977953 ) ) ;
#5602=PLANE ( 'NONE',  #15892 ) ;
#5604=ORIENTED_EDGE ( 'NONE', *, *, #16092, .F. ) ;
#5605=ORIENTED_EDGE ( 'NONE', *, *, #8285, .F. ) ;
#5612=AXIS2_PLACEMENT_3D ( 'NONE', #21252, #5672, #19371 ) ;
#5630=LINE ( 'NONE', #12056, #7479 ) ;
#5631=CARTESIAN_POINT ( 'NONE',  ( 59.52193197173441774, 32.54502000000000095, -3.260183413611184911 ) ) ;
#5632=CARTESIAN_POINT ( 'NONE',  ( 61.04701390398659555, 34.52875999999999834, -15.15157976445104993 ) ) ;
#5633=CARTESIAN_POINT ( 'NONE',  ( 32.17043356788648367, 2.586003464000000029, -17.71146456218788146 ) ) ;
#5634=ORIENTED_EDGE ( 'NONE', *, *, #16460, .F. ) ;
#5646=CIRCLE ( 'NONE', #20449, 0.5080000000000006732 ) ;
#5652=AXIS2_PLACEMENT_3D ( 'NONE', #1773, #1456, #9968 ) ;
#5663=CIRCLE ( 'NONE', #17312, 0.5079999999999973426 ) ;
#5668=LINE ( 'NONE', #3797, #2529 ) ;
#5672=DIRECTION ( 'NONE',  ( -0.9987059298363656357, 0.000000000000000000, -0.05085730733808393328 ) ) ;
#5677=CARTESIAN_POINT ( 'NONE',  ( 52.69799253609296130, -5.166360000000003616, -16.33142188479335744 ) ) ;
#5678=ORIENTED_EDGE ( 'NONE', *, *, #1777, .T. ) ;
#5690=VERTEX_POINT ( 'NONE', #5631 ) ;
#5693=CIRCLE ( 'NONE', #3219, 30.16249999999998721 ) ;
#5694=CARTESIAN_POINT ( 'NONE',  ( 52.43047507149418607, 39.68795354937129360, -17.37982868320523977 ) ) ;
#5695=ORIENTED_EDGE ( 'NONE', *, *, #4747, .T. ) ;
#5700=FACE_OUTER_BOUND ( 'NONE', #14500, .T. ) ;
#5705=CARTESIAN_POINT ( 'NONE',  ( 42.79471501377724252, -1.983739999999999837, 5.049205022181460834 ) ) ;
#5712=CARTESIAN_POINT ( 'NONE',  ( 46.03750000000000142, 34.52875999999999834, -10.31874999999999964 ) ) ;
#5718=CARTESIAN_POINT ( 'NONE',  ( 38.96848998618624904, -7.547609999999999708, -3.934807454472129429 ) ) ;
#5720=CIRCLE ( 'NONE', #20894, 1.190625000000000711 ) ;
#5721=ORIENTED_EDGE ( 'NONE', *, *, #8042, .T. ) ;
#5730=FACE_OUTER_BOUND ( 'NONE', #20356, .T. ) ;
#5731=ORIENTED_EDGE ( 'NONE', *, *, #13671, .T. ) ;
#5734=B_SPLINE_CURVE_WITH_KNOTS ( 'NONE', 3,
 ( #4224, #9410, #9302, #12745 ),
 .UNSPECIFIED., .F., .F.,
 ( 4, 4 ),
 ( 0.008329792089495299118, 0.009162609743145318231 ),
 .UNSPECIFIED. ) ;
#5735=EDGE_LOOP ( 'NONE', ( #5605, #1849, #6831, #6233 ) ) ;
#5738=CIRCLE ( 'NONE', #13526, 4.365624999999999645 ) ;
#5743=DIRECTION ( 'NONE',  ( 0.9724402360367340181, 0.000000000000000000, -0.2331522835762512846 ) ) ;
#5745=CARTESIAN_POINT ( 'NONE',  ( 37.51913901087312553, 42.06303499999999929, -14.58057485080488114 ) ) ;
#5749=CARTESIAN_POINT ( 'NONE',  ( 41.45112526417833010, -1.983739999999999837, 7.778260066349530710 ) ) ;
#5753=ORIENTED_EDGE ( 'NONE', *, *, #17894, .T. ) ;
#5754=ORIENTED_EDGE ( 'NONE', *, *, #9943, .T. ) ;
#5760=ORIENTED_EDGE ( 'NONE', *, *, #4364, .F. ) ;
#5775=AXIS2_PLACEMENT_3D ( 'NONE', #2450, #18427, #5866 ) ;
#5776=DIRECTION ( 'NONE',  ( 0.6702301885068630005, 0.000000000000000000, 0.7421532822901580895 ) ) ;
#5788=DIRECTION ( 'NONE',  ( 0.2064631973582987667, 0.000000000000000000, -0.9784543669157944601 ) ) ;
#5794=CARTESIAN_POINT ( 'NONE',  ( 50.62387473582167274, 0.000000000000000000, -28.41576006634952734 ) ) ;
#5795=CIRCLE ( 'NONE', #17815, 0.5079999999999963434 ) ;
#5800=FACE_OUTER_BOUND ( 'NONE', #8300, .T. ) ;
#5808=CIRCLE ( 'NONE', #9333, 0.5080000000000011173 ) ;
#5814=DIRECTION ( 'NONE',  ( -0.8943161143440100380, 0.000000000000000000, -0.4474356798743612806 ) ) ;
#5816=CARTESIAN_POINT ( 'NONE',  ( 34.38097451710952868, 32.54502000000000095, 0.2081255904771098786 ) ) ;
#5818=CARTESIAN_POINT ( 'NONE',  ( 39.38301085650398647, -7.397690232646351838, -3.502300841008181287 ) ) ;
#5819=EDGE_LOOP ( 'NONE', ( #11774, #18519, #5452, #7970 ) ) ;
#5823=LINE ( 'NONE', #17548, #806 ) ;
#5824=DIRECTION ( 'NONE',  ( -0.2064631973582987667, 0.000000000000000000, 0.9784543669157944601 ) ) ;
#5826=DIRECTION ( 'NONE',  ( -0.6702301885068630005, 0.000000000000000000, -0.7421532822901579785 ) ) ;
#5835=ORIENTED_EDGE ( 'NONE', *, *, #9023, .T. ) ;
#5837=ORIENTED_EDGE ( 'NONE', *, *, #11133, .F. ) ;
#5838=EDGE_CURVE ( 'NONE', #1190, #2509, #18432, .T. ) ;
#5857=VERTEX_POINT ( 'NONE', #21319 ) ;
#5862=CARTESIAN_POINT ( 'NONE',  ( 43.49132289107146931, 34.52875999999999834, 4.686923926377883021 ) ) ;
#5866=DIRECTION ( 'NONE',  ( 0.9724402360367340181, 0.000000000000000000, -0.2331522835762512846 ) ) ;
#5868=LINE ( 'NONE', #12632, #7038 ) ;
#5880=ADVANCED_FACE ( 'NONE', ( #17906 ), #19982, .T. ) ;
#5882=ORIENTED_EDGE ( 'NONE', *, *, #14010, .T. ) ;
#5889=VECTOR ( 'NONE', #8278, 1000.000000000000000 ) ;
#5900=CARTESIAN_POINT ( 'NONE',  ( 52.96420052373725440, 32.54502000000000095, 7.017842122255405712 ) ) ;
#5904=CARTESIAN_POINT ( 'NONE',  ( 52.32428405346736611, 39.49694501955431036, -17.47444899681294217 ) ) ;
#5905=ORIENTED_EDGE ( 'NONE', *, *, #3028, .F. ) ;
#5907=CARTESIAN_POINT ( 'NONE',  ( 53.10322573897614973, 37.69740999999999786, -16.70632925929051638 ) ) ;
#5910=DIRECTION ( 'NONE',  ( 0.000000000000000000, 1.000000000000000000, 0.000000000000000000 ) ) ;
#5911=VERTEX_POINT ( 'NONE', #10475 ) ;
#5912=DIRECTION ( 'NONE',  ( 0.000000000000000000, 1.000000000000000000, 0.000000000000000000 ) ) ;
#5913=CARTESIAN_POINT ( 'NONE',  ( 39.47917727842295932, -7.309119366952678831, -3.410336071361241839 ) ) ;
#5914=VERTEX_POINT ( 'NONE', #15144 ) ;
#5915=CARTESIAN_POINT ( 'NONE',  ( 38.96848998618624904, 37.69740999999999786, -3.934807454472129429 ) ) ;
#5938=AXIS2_PLACEMENT_3D ( 'NONE', #20588, #371, #18504 ) ;
#5941=CARTESIAN_POINT ( 'NONE',  ( 39.80287034594652340, 38.26567781475652907, -3.117403183957448309 ) ) ;
#5942=FACE_OUTER_BOUND ( 'NONE', #20778, .T. ) ;
#5943=CARTESIAN_POINT ( 'NONE',  ( 31.05388211198297554, -1.983739999999999837, -15.23127950648024331 ) ) ;
#5946=ORIENTED_EDGE ( 'NONE', *, *, #21824, .F. ) ;
#5947=DIRECTION ( 'NONE',  ( 0.000000000000000000, -1.000000000000000000, -0.000000000000000000 ) ) ;
#5963=FACE_OUTER_BOUND ( 'NONE', #9662, .T. ) ;
#5965=CARTESIAN_POINT ( 'NONE',  ( 54.61912012054379062, -6.356984999999999886, -13.79062155615056362 ) ) ;
#5966=ADVANCED_FACE ( 'NONE', ( #6834, #18759 ), #3740, .T. ) ;
#5969=CARTESIAN_POINT ( 'NONE',  ( 50.29383871662588490, 34.52875999999999834, -28.02957329025317179 ) ) ;
#5973=EDGE_CURVE ( 'NONE', #15045, #7695, #18546, .T. ) ;
#5977=DIRECTION ( 'NONE',  ( 0.6702301885068628895, 0.000000000000000000, 0.7421532822901579785 ) ) ;
#5982=AXIS2_PLACEMENT_3D ( 'NONE', #13585, #18751, #13471 ) ;
#5985=ORIENTED_EDGE ( 'NONE', *, *, #2025, .F. ) ;
#5986=AXIS2_PLACEMENT_3D ( 'NONE', #15276, #13290, #11608 ) ;
#5993=AXIS2_PLACEMENT_3D ( 'NONE', #940, #2608, #5814 ) ;
#5994=DIRECTION ( 'NONE',  ( 0.8667647648559581031, 0.000000000000000000, 0.4987171968201974948 ) ) ;
#5996=ORIENTED_EDGE ( 'NONE', *, *, #8406, .T. ) ;
#6002=VECTOR ( 'NONE', #7334, 1000.000000000000000 ) ;
#6006=CYLINDRICAL_SURFACE ( 'NONE', #7923, 30.16250000000000142 ) ;
#6007=DIRECTION ( 'NONE',  ( 0.000000000000000000, -1.000000000000000000, -0.000000000000000000 ) ) ;
#6010=AXIS2_PLACEMENT_3D ( 'NONE', #3447, #10180, #18477 ) ;
#6013=ORIENTED_EDGE ( 'NONE', *, *, #2901, .T. ) ;
#6018=CIRCLE ( 'NONE', #20798, 0.7950199999999988387 ) ;
#6025=EDGE_CURVE ( 'NONE', #2096, #17518, #21175, .T. ) ;
#6026=CIRCLE ( 'NONE', #20149, 0.7950199999999993938 ) ;
#6027=EDGE_CURVE ( 'NONE', #16499, #3464, #2400, .T. ) ;
#6031=VERTEX_POINT ( 'NONE', #11230 ) ;
#6033=VECTOR ( 'NONE', #21633, 1000.000000000000000 ) ;
#6034=CARTESIAN_POINT ( 'NONE',  ( 37.51913901087312553, 42.06303499999999929, -14.58057485080488114 ) ) ;
#6035=CIRCLE ( 'NONE', #10637, 1.190625000000001155 ) ;
#6039=DIRECTION ( 'NONE',  ( 0.05085730733808393328, 0.000000000000000000, -0.9987059298363656357 ) ) ;
#6041=EDGE_LOOP ( 'NONE', ( #17010, #331, #2295, #9332 ) ) ;
#6043=CARTESIAN_POINT ( 'NONE',  ( 39.93069333242032570, 38.88803500000010160, -3.008993689095761148 ) ) ;
#6045=CARTESIAN_POINT ( 'NONE',  ( 48.58367710892853353, 34.52875999999999834, -25.32442392637788231 ) ) ;
#6046=EDGE_LOOP ( 'NONE', ( #14554, #19961 ) ) ;
#6048=ORIENTED_EDGE ( 'NONE', *, *, #1833, .F. ) ;
#6053=EDGE_CURVE ( 'NONE', #17565, #13169, #7370, .T. ) ;
#6055=VECTOR ( 'NONE', #12866, 1000.000000000000114 ) ;
#6064=DIRECTION ( 'NONE',  ( 0.9784543669157944601, -0.000000000000000000, 0.2064631973582987945 ) ) ;
#6067=DIRECTION ( 'NONE',  ( -0.9987059298363657467, 0.000000000000000000, -0.05085730733808445370 ) ) ;
#6075=ORIENTED_EDGE ( 'NONE', *, *, #1271, .F. ) ;
#6079=CARTESIAN_POINT ( 'NONE',  ( 43.49132289107146931, 0.000000000000000000, 4.686923926377883021 ) ) ;
#6082=VECTOR ( 'NONE', #11868, 1000.000000000000000 ) ;
#6085=EDGE_CURVE ( 'NONE', #21393, #10995, #6026, .T. ) ;
#6086=CIRCLE ( 'NONE', #12102, 30.16249999999998366 ) ;
#6087=DIRECTION ( 'NONE',  ( 0.000000000000000000, 1.000000000000000000, 0.000000000000000000 ) ) ;
#6092=CARTESIAN_POINT ( 'NONE',  ( 49.72033008250774344, 34.52875999999999124, -2.687827786179598277 ) ) ;
#6098=CARTESIAN_POINT ( 'NONE',  ( 53.46798503507454825, 0.000000000000000000, 6.304111036318381878 ) ) ;
#6101=ORIENTED_EDGE ( 'NONE', *, *, #14696, .F. ) ;
#6111=EDGE_CURVE ( 'NONE', #15942, #16009, #21617, .T. ) ;
#6112=DIRECTION ( 'NONE',  ( 0.4987171968201936645, 0.000000000000000000, -0.8667647648559603235 ) ) ;
#6134=LINE ( 'NONE', #4483, #11649 ) ;
#6135=ORIENTED_EDGE ( 'NONE', *, *, #13900, .T. ) ;
#6136=( NAMED_UNIT ( * ) SI_UNIT ( $, .STERADIAN. ) SOLID_ANGLE_UNIT ( ) );
#6139=ORIENTED_EDGE ( 'NONE', *, *, #7483, .F. ) ;
#6145=EDGE_LOOP ( 'NONE', ( #13443, #13119, #314, #6996 ) ) ;
#6149=CIRCLE ( 'NONE', #16752, 0.5079999999999984528 ) ;
#6151=CARTESIAN_POINT ( 'NONE',  ( 38.95866807045890567, -7.547549837578408471, -3.945694591016585928 ) ) ;
#6156=VECTOR ( 'NONE', #16143, 1000.000000000000114 ) ;
#6168=AXIS2_PLACEMENT_3D ( 'NONE', #923, #2914, #21141 ) ;
#6170=ORIENTED_EDGE ( 'NONE', *, *, #12226, .T. ) ;
#6173=DIRECTION ( 'NONE',  ( 0.000000000000000000, 1.000000000000000000, 0.000000000000000000 ) ) ;
#6174=FACE_OUTER_BOUND ( 'NONE', #11039, .T. ) ;
#6177=ORIENTED_EDGE ( 'NONE', *, *, #4747, .F. ) ;
#6181=CARTESIAN_POINT ( 'NONE',  ( 47.80475250345343596, 38.88803500000000213, -11.91473563638196786 ) ) ;
#6192=FACE_OUTER_BOUND ( 'NONE', #3880, .T. ) ;
#6205=CARTESIAN_POINT ( 'NONE',  ( 49.72033008250774344, -1.983739999999999837, -2.687827786179598277 ) ) ;
#6219=CARTESIAN_POINT ( 'NONE',  ( 44.27024749654656688, -7.547609999999999708, -8.722764363618033201 ) ) ;
#6224=DIRECTION ( 'NONE',  ( -0.9724402360367336851, 0.000000000000000000, 0.2331522835762537549 ) ) ;
#6228=CARTESIAN_POINT ( 'NONE',  ( 64.19677489640052670, 34.52875999999999834, -11.74367670905533423 ) ) ;
#6229=ADVANCED_FACE ( 'NONE', ( #10009 ), #1913, .F. ) ;
#6231=DIRECTION ( 'NONE',  ( 0.6496772031432432870, 0.000000000000000000, -0.7602101891687411683 ) ) ;
#6233=ORIENTED_EDGE ( 'NONE', *, *, #9501, .T. ) ;
#6235=CARTESIAN_POINT ( 'NONE',  ( 44.27024749654656688, 40.07865999999999929, -8.722764363618033201 ) ) ;
#6249=CARTESIAN_POINT ( 'NONE',  ( 38.76233322772463197, 40.04759419886305949, -4.169083009079019853 ) ) ;
#6252=FACE_OUTER_BOUND ( 'NONE', #21429, .T. ) ;
#6258=CARTESIAN_POINT ( 'NONE',  ( 30.50878709810603340, -4.569743463999999200, -19.83971405306587954 ) ) ;
#6261=PLANE ( 'NONE',  #21860 ) ;
#6263=CARTESIAN_POINT ( 'NONE',  ( 46.03750000000000142, 0.000000000000000000, -10.31874999999999964 ) ) ;
#6264=EDGE_LOOP ( 'NONE', ( #14536, #11321, #2359, #2878, #7202, #6870, #531, #8223, #12958, #10461, #14034, #189, #1680, #3502, #19195, #11540, #16282, #297, #6592, #4059, #2387, #11791, #16453, #11632, #21217, #19822, #7471, #21064, #9039, #3214, #15807, #4728, #5187, #2527, #9558, #3862, #6288, #41, #4659, #19587 ) ) ;
#6277=ORIENTED_EDGE ( 'NONE', *, *, #10409, .T. ) ;
#6284=ORIENTED_EDGE ( 'NONE', *, *, #16958, .F. ) ;
#6286=CARTESIAN_POINT ( 'NONE',  ( 41.71184157647478230, 38.88803500000000213, -2.134205101306931862 ) ) ;
#6288=ORIENTED_EDGE ( 'NONE', *, *, #11325, .T. ) ;
#6295=ADVANCED_FACE ( 'NONE', ( #11550 ), #1482, .T. ) ;
#6300=CYLINDRICAL_SURFACE ( 'NONE', #20814, 0.5079999999999996740 ) ;
#6304=EDGE_LOOP ( 'NONE', ( #3709, #2071, #18573, #7081 ) ) ;
#6307=CARTESIAN_POINT ( 'NONE',  ( 50.62387473582167274, -1.983739999999999837, -28.41576006634952734 ) ) ;
#6309=DIRECTION ( 'NONE',  ( 0.4987171968201928873, 0.000000000000000000, -0.8667647648559606566 ) ) ;
#6311=CARTESIAN_POINT ( 'NONE',  ( 55.33978576324753362, 0.000000000000000000, -23.05096232720518756 ) ) ;
#6313=CIRCLE ( 'NONE', #14106, 9.525000000000002132 ) ;
#6318=CYLINDRICAL_SURFACE ( 'NONE', #12698, 9.524999999999998579 ) ;
#6329=VECTOR ( 'NONE', #16215, 1000.000000000000114 ) ;
#6330=FACE_OUTER_BOUND ( 'NONE', #17771, .T. ) ;
#6332=DIRECTION ( 'NONE',  ( -0.7421532822901579785, 0.000000000000000000, 0.6702301885068630005 ) ) ;
#6334=DIRECTION ( 'NONE',  ( 0.000000000000000000, 1.000000000000000000, 0.000000000000000000 ) ) ;
#6338=CARTESIAN_POINT ( 'NONE',  ( 53.69636427252483202, 38.88803500000000213, -18.48840734645144224 ) ) ;
#6342=CARTESIAN_POINT ( 'NONE',  ( 52.22364792556211910, 38.56942770589630953, -17.56175453227104200 ) ) ;
#6345=CARTESIAN_POINT ( 'NONE',  ( 38.60701496492545459, 32.54502000000000095, -26.94161103631838472 ) ) ;
#6361=CARTESIAN_POINT ( 'NONE',  ( 42.27821610176829381, -1.983739999999999837, 7.496956594510385763 ) ) ;
#6362=LINE ( 'NONE', #15672, #4249 ) ;
#6363=EDGE_LOOP ( 'NONE', ( #7392, #13518, #4896, #17810 ) ) ;
#6368=ORIENTED_EDGE ( 'NONE', *, *, #18799, .F. ) ;
#6369=EDGE_LOOP ( 'NONE', ( #17817, #7925, #16660, #13328 ) ) ;
#6372=CARTESIAN_POINT ( 'NONE',  ( 37.51913901087312553, 42.06303499999999929, -14.58057485080488114 ) ) ;
#6383=ORIENTED_EDGE ( 'NONE', *, *, #964, .T. ) ;
#6384=ADVANCED_FACE ( 'NONE', ( #5021 ), #11776, .T. ) ;
#6387=DIRECTION ( 'NONE',  ( 0.000000000000000000, 1.000000000000000000, 0.000000000000000000 ) ) ;
#6393=ORIENTED_EDGE ( 'NONE', *, *, #18942, .T. ) ;
#6394=VECTOR ( 'NONE', #5247, 1000.000000000000000 ) ;
#6398=CARTESIAN_POINT ( 'NONE',  ( 53.10651001381376091, 37.69740999999999786, -16.70269254552787075 ) ) ;
#6400=ORIENTED_EDGE ( 'NONE', *, *, #2874, .F. ) ;
#6402=CARTESIAN_POINT ( 'NONE',  ( 40.38185354615648492, 38.88803500000000213, -3.606915520851464052 ) ) ;
#6405=VECTOR ( 'NONE', #15971, 1000.000000000000000 ) ;
#6406=ORIENTED_EDGE ( 'NONE', *, *, #2312, .F. ) ;
#6410=AXIS2_PLACEMENT_3D ( 'NONE', #5438, #19265, #13990 ) ;
#6417=DIRECTION ( 'NONE',  ( 0.8667647648559581031, 0.000000000000000000, 0.4987171968201974948 ) ) ;
#6421=CARTESIAN_POINT ( 'NONE',  ( 53.92979111630407374, -6.356984999999459873, -15.65141968182990162 ) ) ;
#6433=ADVANCED_FACE ( 'NONE', ( #2361 ), #5336, .T. ) ;
#6444=DIRECTION ( 'NONE',  ( 0.7421532822901579785, 0.000000000000000000, -0.6702301885068630005 ) ) ;
#6450=CARTESIAN_POINT ( 'NONE',  ( 54.55586098912687731, -9.531985000000000596, -6.056925149195119040 ) ) ;
#6452=CARTESIAN_POINT ( 'NONE',  ( 39.72822375471606193, 39.64629009929521430, -3.182007191425374693 ) ) ;
#6458=CARTESIAN_POINT ( 'NONE',  ( 57.35354854712898742, 34.52875999999999834, -21.22263945788050776 ) ) ;
#6467=CYLINDRICAL_SURFACE ( 'NONE', #8814, 30.16250000000000142 ) ;
#6471=ORIENTED_EDGE ( 'NONE', *, *, #4405, .T. ) ;
#6473=CARTESIAN_POINT ( 'NONE',  ( 53.10651001381376091, -7.547610000000002373, -16.70269254552787075 ) ) ;
#6476=VERTEX_POINT ( 'NONE', #14104 ) ;
#6479=CARTESIAN_POINT ( 'NONE',  ( 42.94469661997857912, 0.000000000000000000, -18.48251861828712705 ) ) ;
#6484=VERTEX_POINT ( 'NONE', #20586 ) ;
#6493=DIRECTION ( 'NONE',  ( 0.3542738219355897056, 0.000000000000000000, 0.9351417320872542627 ) ) ;
#6496=CIRCLE ( 'NONE', #16042, 0.5080000000000012284 ) ;
#6497=ORIENTED_EDGE ( 'NONE', *, *, #14126, .F. ) ;
#6506=CARTESIAN_POINT ( 'NONE',  ( 30.50878709810603340, 0.000000000000000000, -19.83971405306587954 ) ) ;
#6510=FACE_OUTER_BOUND ( 'NONE', #6944, .T. ) ;
#6514=CARTESIAN_POINT ( 'NONE',  ( 39.88301061098722755, 34.52875999999999834, -24.08706006053352411 ) ) ;
#6523=VECTOR ( 'NONE', #1890, 1000.000000000000114 ) ;
#6532=DIRECTION ( 'NONE',  ( 0.9784543669157947932, 0.000000000000000000, 0.2064631973582977953 ) ) ;
#6538=DIRECTION ( 'NONE',  ( 0.000000000000000000, -1.000000000000000000, 0.000000000000000000 ) ) ;
#6540=VECTOR ( 'NONE', #16786, 1000.000000000000114 ) ;
#6546=ORIENTED_EDGE ( 'NONE', *, *, #13409, .F. ) ;
#6563=CARTESIAN_POINT ( 'NONE',  ( 55.27198911326564001, -1.983739999999999837, 2.462719476673013830 ) ) ;
#6564=ORIENTED_EDGE ( 'NONE', *, *, #12132, .T. ) ;
#6567=DIRECTION ( 'NONE',  ( 0.000000000000000000, 1.000000000000000000, -0.000000000000000000 ) ) ;
#6569=CARTESIAN_POINT ( 'NONE',  ( 35.15748561355322011, 32.54502000000000095, 0.3244898641346534163 ) ) ;
#6572=ORIENTED_EDGE ( 'NONE', *, *, #18123, .T. ) ;
#6584=EDGE_CURVE ( 'NONE', #15435, #2625, #19598, .T. ) ;
#6587=DIRECTION ( 'NONE',  ( 0.000000000000000000, 1.000000000000000000, 0.000000000000000000 ) ) ;
#6592=ORIENTED_EDGE ( 'NONE', *, *, #7074, .T. ) ;
#6594=DIRECTION ( 'NONE',  ( 0.000000000000000000, -1.000000000000000000, -0.000000000000000000 ) ) ;
#6597=VERTEX_POINT ( 'NONE', #3021 ) ;
#6601=DIRECTION ( 'NONE',  ( 0.000000000000000000, 1.000000000000000000, 0.000000000000000000 ) ) ;
#6605=CARTESIAN_POINT ( 'NONE',  ( 30.47347900023190803, 37.11476346399999926, -8.148724574017967015 ) ) ;
#6606=CARTESIAN_POINT ( 'NONE',  ( 34.72145145287101542, 32.54502000000000095, 0.5851394578805096947 ) ) ;
#6611=DIRECTION ( 'NONE',  ( 0.000000000000000000, -1.000000000000000000, -0.000000000000000000 ) ) ;
#6615=CARTESIAN_POINT ( 'NONE',  ( 38.54095024924464497, 38.88803500000000213, -2.295677052105690841 ) ) ;
#6617=ORIENTED_EDGE ( 'NONE', *, *, #18579, .T. ) ;
#6623=CIRCLE ( 'NONE', #2026, 0.5080000000000022276 ) ;
#6631=DIRECTION ( 'NONE',  ( 0.7421532822901579785, -0.000000000000000000, -0.6702301885068630005 ) ) ;
#6643=EDGE_CURVE ( 'NONE', #18042, #3414, #8829, .T. ) ;
#6646=ADVANCED_FACE ( 'NONE', ( #21693 ), #4883, .T. ) ;
#6647=CARTESIAN_POINT ( 'NONE',  ( 49.79678389823170903, 32.54502000000000095, -28.13445659451038594 ) ) ;
#6654=CARTESIAN_POINT ( 'NONE',  ( 53.69636427252483202, 38.88803500000000213, -18.48840734645144224 ) ) ;
#6656=CARTESIAN_POINT ( 'NONE',  ( 52.96420052373725440, -1.983739999999999837, 7.017842122255405712 ) ) ;
#6661=DIRECTION ( 'NONE',  ( 0.000000000000000000, -1.000000000000000000, -0.000000000000000000 ) ) ;
#6675=DIRECTION ( 'NONE',  ( 0.000000000000000000, 1.000000000000000000, 0.000000000000000000 ) ) ;
#6676=CIRCLE ( 'NONE', #15522, 0.5080000000000014504 ) ;
#6683=EDGE_CURVE ( 'NONE', #1698, #8377, #13797, .T. ) ;
#6687=CARTESIAN_POINT ( 'NONE',  ( 38.96848998618624904, 37.69740999999999786, -3.934807454472129429 ) ) ;
#6695=ORIENTED_EDGE ( 'NONE', *, *, #10352, .T. ) ;
#6696=DIRECTION ( 'NONE',  ( 0.000000000000000000, -1.000000000000000000, -0.000000000000000000 ) ) ;
#6715=CARTESIAN_POINT ( 'NONE',  ( 42.27821610176829381, 0.000000000000000000, 7.496956594510385763 ) ) ;
#6716=AXIS2_PLACEMENT_3D ( 'NONE', #18518, #18617, #20372 ) ;
#6725=VECTOR ( 'NONE', #11063, 1000.000000000000000 ) ;
#6733=AXIS2_PLACEMENT_3D ( 'NONE', #6986, #3793, #5118 ) ;
#6736=CIRCLE ( 'NONE', #7441, 30.16249999999998721 ) ;
#6738=DIRECTION ( 'NONE',  ( 0.000000000000000000, 1.000000000000000000, 0.000000000000000000 ) ) ;
#6745=DIRECTION ( 'NONE',  ( 0.000000000000000000, 1.000000000000000000, 0.000000000000000000 ) ) ;
#6748=EDGE_LOOP ( 'NONE', ( #18825, #14326, #21435, #8986 ) ) ;
#6751=ORIENTED_EDGE ( 'NONE', *, *, #12132, .F. ) ;
#6757=DIRECTION ( 'NONE',  ( 0.000000000000000000, 1.000000000000000000, 0.000000000000000000 ) ) ;
#6758=DIRECTION ( 'NONE',  ( -0.8583349619704310207, 0.000000000000000000, 0.5130897514657826175 ) ) ;
#6770=CYLINDRICAL_SURFACE ( 'NONE', #2854, 0.7950199999999982836 ) ;
#6771=AXIS2_PLACEMENT_3D ( 'NONE', #14822, #4311, #17806 ) ;
#6772=EDGE_LOOP ( 'NONE', ( #6820, #689, #17986, #3496 ) ) ;
#6776=CYLINDRICAL_SURFACE ( 'NONE', #1640, 1.190624999999997824 ) ;
#6777=VERTEX_POINT ( 'NONE', #14861 ) ;
#6784=CARTESIAN_POINT ( 'NONE',  ( 27.87822510359947614, 34.52875999999999834, -8.893823290944665061 ) ) ;
#6800=AXIS2_PLACEMENT_3D ( 'NONE', #2003, #7100, #13531 ) ;
#6803=ORIENTED_EDGE ( 'NONE', *, *, #15440, .T. ) ;
#6810=VECTOR ( 'NONE', #19023, 1000.000000000000000 ) ;
#6811=EDGE_CURVE ( 'NONE', #17559, #2599, #10612, .T. ) ;
#6817=ORIENTED_EDGE ( 'NONE', *, *, #18997, .T. ) ;
#6820=ORIENTED_EDGE ( 'NONE', *, *, #261, .T. ) ;
#6826=CARTESIAN_POINT ( 'NONE',  ( 64.19677489640052670, 0.000000000000000000, -11.74367670905533423 ) ) ;
#6831=ORIENTED_EDGE ( 'NONE', *, *, #13897, .F. ) ;
#6832=DIRECTION ( 'NONE',  ( 0.000000000000000000, 1.000000000000000000, 0.000000000000000000 ) ) ;
#6834=FACE_BOUND ( 'NONE', #21681, .T. ) ;
#6839=ORIENTED_EDGE ( 'NONE', *, *, #114, .F. ) ;
#6843=FACE_OUTER_BOUND ( 'NONE', #11614, .T. ) ;
#6855=EDGE_CURVE ( 'NONE', #16499, #14487, #20463, .T. ) ;
#6860=LINE ( 'NONE', #6960, #14211 ) ;
#6861=DIRECTION ( 'NONE',  ( 0.000000000000000000, 1.000000000000000000, 0.000000000000000000 ) ) ;
#6870=ORIENTED_EDGE ( 'NONE', *, *, #6643, .F. ) ;
#6877=CIRCLE ( 'NONE', #13549, 1.984375000000000000 ) ;
#6907=ADVANCED_BREP_SHAPE_REPRESENTATION ( '', ( #13288, #2234 ), #5057 ) ;
#6909=CARTESIAN_POINT ( 'NONE',  ( 52.44708915697334106, 0.000000000000000000, 4.020247972991190188 ) ) ;
#6917=DIRECTION ( 'NONE',  ( 0.000000000000000000, 1.000000000000000000, 0.000000000000000000 ) ) ;
#6918=ORIENTED_EDGE ( 'NONE', *, *, #1288, .F. ) ;
#6920=VERTEX_POINT ( 'NONE', #12182 ) ;
#6924=VERTEX_POINT ( 'NONE', #229 ) ;
#6928=DIRECTION ( 'NONE',  ( 0.9129422336036140395, 0.000000000000000000, -0.4080888115384250225 ) ) ;
#6929=DIRECTION ( 'NONE',  ( 0.000000000000000000, 1.000000000000000000, -0.000000000000000000 ) ) ;
#6930=DIRECTION ( 'NONE',  ( 0.8583349619704303546, 0.000000000000000000, -0.5130897514657839498 ) ) ;
#6940=ORIENTED_EDGE ( 'NONE', *, *, #9616, .T. ) ;
#6944=EDGE_LOOP ( 'NONE', ( #148, #12725, #19644, #4954 ) ) ;
#6947=CIRCLE ( 'NONE', #21778, 0.5080000000000023386 ) ;
#6952=ADVANCED_FACE ( 'NONE', ( #4324 ), #12618, .T. ) ;
#6954=CARTESIAN_POINT ( 'NONE',  ( 61.09555596642878328, 34.52875999999999834, -12.53419992421059348 ) ) ;
#6960=CARTESIAN_POINT ( 'NONE',  ( 38.82016491058538321, -9.531985000000000596, -14.75770094105646812 ) ) ;
#6961=DIRECTION ( 'NONE',  ( 0.9724402360367340181, 0.000000000000000000, -0.2331522835762512846 ) ) ;
#6965=DIRECTION ( 'NONE',  ( 0.000000000000000000, 1.000000000000000000, 0.000000000000000000 ) ) ;
#6975=ADVANCED_FACE ( 'NONE', ( #16273 ), #2665, .T. ) ;
#6976=EDGE_CURVE ( 'NONE', #4294, #5857, #19341, .T. ) ;
#6986=CARTESIAN_POINT ( 'NONE',  ( 39.07078961959606289, 32.54502000000000095, -27.14892015257980162 ) ) ;
#6988=CARTESIAN_POINT ( 'NONE',  ( 59.52193197173441774, 0.000000000000000000, -3.260183413611184911 ) ) ;
#6990=DIRECTION ( 'NONE',  ( 0.000000000000000000, 1.000000000000000000, 0.000000000000000000 ) ) ;
#6996=ORIENTED_EDGE ( 'NONE', *, *, #20699, .F. ) ;
#7000=EDGE_CURVE ( 'NONE', #10564, #20253, #2442, .T. ) ;
#7026=CARTESIAN_POINT ( 'NONE',  ( 61.60152099976809126, 2.586003464000000029, -12.48877542598203405 ) ) ;
#7032=CARTESIAN_POINT ( 'NONE',  ( 36.73521423675246922, -1.983739999999999837, 2.413462327205186497 ) ) ;
#7033=CARTESIAN_POINT ( 'NONE',  ( 53.84486179190094646, -1.983739999999999837, -6.412645463410259872 ) ) ;
#7038=VECTOR ( 'NONE', #11177, 1000.000000000000000 ) ;
#7039=LINE ( 'NONE', #1955, #20579 ) ;
#7040=DIRECTION ( 'NONE',  ( -0.9784543669157944601, 0.000000000000000000, -0.2064631973582987667 ) ) ;
#7047=ORIENTED_EDGE ( 'NONE', *, *, #13582, .F. ) ;
#7055=CARTESIAN_POINT ( 'NONE',  ( 53.84486179190094646, 34.52875999999999834, -6.412645463410259872 ) ) ;
#7063=AXIS2_PLACEMENT_3D ( 'NONE', #4452, #21343, #19680 ) ;
#7065=DIRECTION ( 'NONE',  ( 0.000000000000000000, 1.000000000000000000, 0.000000000000000000 ) ) ;
#7072=DIRECTION ( 'NONE',  ( 0.1060008583745224581, 0.000000000000000000, 0.9943660382494288186 ) ) ;
#7074=EDGE_CURVE ( 'NONE', #15662, #4928, #14531, .T. ) ;
#7078=CIRCLE ( 'NONE', #7063, 0.5080000000000000071 ) ;
#7081=ORIENTED_EDGE ( 'NONE', *, *, #13591, .T. ) ;
#7082=CIRCLE ( 'NONE', #14867, 0.5079999999999984528 ) ;
#7083=ORIENTED_EDGE ( 'NONE', *, *, #19281, .T. ) ;
#7090=CIRCLE ( 'NONE', #11343, 9.525000000000000355 ) ;
#7091=DIRECTION ( 'NONE',  ( 0.05085730733808139364, 0.000000000000000000, -0.9987059298363658577 ) ) ;
#7097=DIRECTION ( 'NONE',  ( 0.4987171968201936645, 0.000000000000000000, -0.8667647648559603235 ) ) ;
#7100=DIRECTION ( 'NONE',  ( -0.000000000000000000, -1.000000000000000000, 0.000000000000000000 ) ) ;
#7110=DIRECTION ( 'NONE',  ( -0.1060008583745200572, 0.000000000000000000, -0.9943660382494290406 ) ) ;
#7113=AXIS2_PLACEMENT_3D ( 'NONE', #10614, #12172, #17248 ) ;
#7119=VECTOR ( 'NONE', #20197, 1000.000000000000000 ) ;
#7122=DIRECTION ( 'NONE',  ( -0.7421532822901562021, 0.000000000000000000, 0.6702301885068651099 ) ) ;
#7124=AXIS2_PLACEMENT_3D ( 'NONE', #12512, #18017, #4099 ) ;
#7136=ADVANCED_FACE ( 'NONE', ( #6192 ), #19667, .T. ) ;
#7143=VECTOR ( 'NONE', #10142, 1000.000000000000000 ) ;
#7153=ORIENTED_EDGE ( 'NONE', *, *, #18805, .F. ) ;
#7157=CYLINDRICAL_SURFACE ( 'NONE', #1146, 0.5079999999999965654 ) ;
#7160=CARTESIAN_POINT ( 'NONE',  ( 38.82016491058538321, 42.06303499999999929, -14.75770094105646812 ) ) ;
#7162=CARTESIAN_POINT ( 'NONE',  ( 42.35466991749225940, 42.06303499999999929, -17.94967221382040279 ) ) ;
#7163=EDGE_CURVE ( 'NONE', #20627, #18152, #7412, .T. ) ;
#7164=DIRECTION ( 'NONE',  ( -0.6702301885068628895, 0.000000000000000000, -0.7421532822901579785 ) ) ;
#7165=AXIS2_PLACEMENT_3D ( 'NONE', #4635, #2654, #19558 ) ;
#7166=EDGE_LOOP ( 'NONE', ( #14920, #7153, #55, #13922 ) ) ;
#7171=VERTEX_POINT ( 'NONE', #9822 ) ;
#7179=CIRCLE ( 'NONE', #1513, 4.365624999999999645 ) ;
#7189=CARTESIAN_POINT ( 'NONE',  ( 38.73876173903332898, -7.523800691136061758, -4.196965627914218899 ) ) ;
#7190=CARTESIAN_POINT ( 'NONE',  ( 39.27728671717661513, 32.54502000000000095, -23.95520057284206672 ) ) ;
#7198=CARTESIAN_POINT ( 'NONE',  ( 39.42154620619601957, -6.356984999999999886, -4.343957374021048423 ) ) ;
#7199=CARTESIAN_POINT ( 'NONE',  ( 53.83440531914143179, -5.732648258448109324, -15.79034767386256988 ) ) ;
#7202=ORIENTED_EDGE ( 'NONE', *, *, #2738, .T. ) ;
#7208=ORIENTED_EDGE ( 'NONE', *, *, #20067, .T. ) ;
#7209=DIRECTION ( 'NONE',  ( -0.7421532822901579785, 0.000000000000000000, 0.6702301885068630005 ) ) ;
#7212=CARTESIAN_POINT ( 'NONE',  ( 64.14292646034530776, 32.54502000000000095, -12.24881465648521939 ) ) ;
#7214=AXIS2_PLACEMENT_3D ( 'NONE', #13720, #1435, #18778 ) ;
#7216=CARTESIAN_POINT ( 'NONE',  ( 59.80894853325292360, -6.356984999999999886, -16.70545285374888778 ) ) ;
#7218=CARTESIAN_POINT ( 'NONE',  ( 39.62791084302666178, -1.983739999999999837, -24.65774797299118859 ) ) ;
#7221=VECTOR ( 'NONE', #20537, 1000.000000000000000 ) ;
#7226=LINE ( 'NONE', #8857, #3988 ) ;
#7228=DIRECTION ( 'NONE',  ( 0.000000000000000000, 1.000000000000000000, 0.000000000000000000 ) ) ;
#7232=DIRECTION ( 'NONE',  ( 0.000000000000000000, -1.000000000000000000, -0.000000000000000000 ) ) ;
#7239=ORIENTED_EDGE ( 'NONE', *, *, #16189, .T. ) ;
#7243=VECTOR ( 'NONE', #18564, 1000.000000000000114 ) ;
#7256=EDGE_LOOP ( 'NONE', ( #16025, #15491, #16691, #4411, #9777, #6695 ) ) ;
#7261=DIRECTION ( 'NONE',  ( 0.000000000000000000, -1.000000000000000000, -0.000000000000000000 ) ) ;
#7271=FACE_OUTER_BOUND ( 'NONE', #19724, .T. ) ;
#7272=DIRECTION ( 'NONE',  ( 0.000000000000000000, -1.000000000000000000, -0.000000000000000000 ) ) ;
#7286=VERTEX_POINT ( 'NONE', #15055 ) ;
#7296=ORIENTED_EDGE ( 'NONE', *, *, #3028, .T. ) ;
#7298=CARTESIAN_POINT ( 'NONE',  ( 64.14292646034530776, 34.52875999999999834, -12.24881465648521939 ) ) ;
#7301=ORIENTED_EDGE ( 'NONE', *, *, #15721, .F. ) ;
#7304=AXIS2_PLACEMENT_3D ( 'NONE', #12511, #774, #12721 ) ;
#7307=ORIENTED_EDGE ( 'NONE', *, *, #11423, .F. ) ;
#7312=CARTESIAN_POINT ( 'NONE',  ( 57.35354854712898742, 0.000000000000000000, -21.22263945788050776 ) ) ;
#7318=AXIS2_PLACEMENT_3D ( 'NONE', #6286, #16694, #9931 ) ;
#7320=FACE_OUTER_BOUND ( 'NONE', #14560, .T. ) ;
#7328=DIRECTION ( 'NONE',  ( 0.000000000000000000, 1.000000000000000000, 0.000000000000000000 ) ) ;
#7331=ADVANCED_FACE ( 'NONE', ( #14948 ), #3098, .F. ) ;
#7334=DIRECTION ( 'NONE',  ( 0.000000000000000000, 1.000000000000000000, -0.000000000000000000 ) ) ;
#7335=VERTEX_POINT ( 'NONE', #19771 ) ;
#7337=CARTESIAN_POINT ( 'NONE',  ( 46.07940063401251507, 34.52875999999999834, -26.08707253294707229 ) ) ;
#7347=DIRECTION ( 'NONE',  ( -0.4080888115384288528, 0.000000000000000000, -0.9129422336036122632 ) ) ;
#7349=LINE ( 'NONE', #5900, #4622 ) ;
#7353=CARTESIAN_POINT ( 'NONE',  ( 39.42154620619643879, -5.166360000000000063, -4.343957374020580353 ) ) ;
#7356=DIRECTION ( 'NONE',  ( 0.000000000000000000, -1.000000000000000000, -0.000000000000000000 ) ) ;
#7368=ORIENTED_EDGE ( 'NONE', *, *, #597, .F. ) ;
#7369=DIRECTION ( 'NONE',  ( 0.05085730733808139364, 0.000000000000000000, -0.9987059298363658577 ) ) ;
#7370=LINE ( 'NONE', #12915, #2197 ) ;
#7380=VERTEX_POINT ( 'NONE', #11926 ) ;
#7386=VERTEX_POINT ( 'NONE', #5816 ) ;
#7391=CIRCLE ( 'NONE', #18674, 0.5080000000000000071 ) ;
#7392=ORIENTED_EDGE ( 'NONE', *, *, #20820, .F. ) ;
#7396=DIRECTION ( 'NONE',  ( 0.000000000000000000, -1.000000000000000000, -0.000000000000000000 ) ) ;
#7403=ORIENTED_EDGE ( 'NONE', *, *, #12212, .T. ) ;
#7405=ORIENTED_EDGE ( 'NONE', *, *, #13057, .T. ) ;
#7412=LINE ( 'NONE', #8062, #21555 ) ;
#7419=CYLINDRICAL_SURFACE ( 'NONE', #3302, 1.190625000000001155 ) ;
#7422=DIRECTION ( 'NONE',  ( 0.000000000000000000, -1.000000000000000000, -0.000000000000000000 ) ) ;
#7426=CIRCLE ( 'NONE', #14504, 0.7950200000000003930 ) ;
#7428=DIRECTION ( 'NONE',  ( -0.000000000000000000, -1.000000000000000000, 0.000000000000000000 ) ) ;
#7441=AXIS2_PLACEMENT_3D ( 'NONE', #10348, #6917, #3495 ) ;
#7452=AXIS2_PLACEMENT_3D ( 'NONE', #3049, #21166, #11335 ) ;
#7453=AXIS2_PLACEMENT_3D ( 'NONE', #3828, #7261, #175 ) ;
#7458=PLANE ( 'NONE',  #19773 ) ;
#7464=DIRECTION ( 'NONE',  ( 0.000000000000000000, -1.000000000000000000, -0.000000000000000000 ) ) ;
#7471=ORIENTED_EDGE ( 'NONE', *, *, #21036, .T. ) ;
#7476=VERTEX_POINT ( 'NONE', #4270 ) ;
#7479=VECTOR ( 'NONE', #8832, 1000.000000000000114 ) ;
#7482=DIRECTION ( 'NONE',  ( -0.3542738219355896501, 0.000000000000000000, -0.9351417320872542627 ) ) ;
#7483=EDGE_CURVE ( 'NONE', #10833, #20627, #9195, .T. ) ;
#7486=CARTESIAN_POINT ( 'NONE',  ( 39.62791084302666178, 0.000000000000000000, -24.65774797299118859 ) ) ;
#7492=DIRECTION ( 'NONE',  ( 0.05085730733808393328, 0.000000000000000000, -0.9987059298363656357 ) ) ;
#7494=VERTEX_POINT ( 'NONE', #12462 ) ;
#7498=ORIENTED_EDGE ( 'NONE', *, *, #19356, .T. ) ;
#7502=ORIENTED_EDGE ( 'NONE', *, *, #6976, .T. ) ;
#7504=VERTEX_POINT ( 'NONE', #1969 ) ;
#7509=ADVANCED_FACE ( 'NONE', ( #20307 ), #14346, .F. ) ;
#7512=DIRECTION ( 'NONE',  ( 0.000000000000000000, -1.000000000000000000, -0.000000000000000000 ) ) ;
#7516=ORIENTED_EDGE ( 'NONE', *, *, #5352, .T. ) ;
#7520=DIRECTION ( 'NONE',  ( 0.000000000000000000, 1.000000000000000000, 0.000000000000000000 ) ) ;
#7523=ORIENTED_EDGE ( 'NONE', *, *, #17168, .T. ) ;
#7524=ORIENTED_EDGE ( 'NONE', *, *, #4449, .T. ) ;
#7529=ORIENTED_EDGE ( 'NONE', *, *, #11602, .T. ) ;
#7536=CARTESIAN_POINT ( 'NONE',  ( 39.00487391864218267, 37.69864044684034354, -3.894748490052650780 ) ) ;
#7544=CIRCLE ( 'NONE', #20224, 0.7950199999999993938 ) ;
#7547=CARTESIAN_POINT ( 'NONE',  ( 52.96420052373725440, 32.54502000000000095, 7.017842122255405712 ) ) ;
#7553=ORIENTED_EDGE ( 'NONE', *, *, #18555, .F. ) ;
#7555=LINE ( 'NONE', #5549, #11006 ) ;
#7558=EDGE_LOOP ( 'NONE', ( #14156, #4502, #6471 ) ) ;
#7560=CARTESIAN_POINT ( 'NONE',  ( 57.23009918853844624, 0.000000000000000000, -20.42665903041912401 ) ) ;
#7561=VECTOR ( 'NONE', #20679, 1000.000000000000114 ) ;
#7567=VECTOR ( 'NONE', #6173, 1000.000000000000000 ) ;
#7570=CARTESIAN_POINT ( 'NONE',  ( 53.35709526732357233, -7.529133977686723433, -16.41569776986803930 ) ) ;
#7575=CIRCLE ( 'NONE', #9680, 0.5079999999999996740 ) ;
#7587=CARTESIAN_POINT ( 'NONE',  ( 38.96848998618624904, -5.166360000000000063, -3.934807454472129429 ) ) ;
#7588=VERTEX_POINT ( 'NONE', #12908 ) ;
#7590=EDGE_CURVE ( 'NONE', #19114, #9035, #9563, .T. ) ;
#7597=EDGE_LOOP ( 'NONE', ( #18186, #13151, #16349, #6817 ) ) ;
#7598=CARTESIAN_POINT ( 'NONE',  ( 49.13030338002142372, 109.3223030719999969, -2.154981381712871791 ) ) ;
#7599=CARTESIAN_POINT ( 'NONE',  ( 39.11241740126524746, -7.547728945059590799, -4.078053966296677935 ) ) ;
#7600=EDGE_LOOP ( 'NONE', ( #20959, #11676, #3016, #6406, #3970 ) ) ;
#7605=EDGE_LOOP ( 'NONE', ( #11132, #20151, #9309, #19548 ) ) ;
#7610=AXIS2_PLACEMENT_3D ( 'NONE', #18273, #13215, #13105 ) ;
#7611=EDGE_CURVE ( 'NONE', #3414, #3770, #14890, .T. ) ;
#7620=EDGE_LOOP ( 'NONE', ( #2836, #11792, #1234, #5025 ) ) ;
#7628=DIRECTION ( 'NONE',  ( -0.8583349619704301325, 0.000000000000000000, 0.5130897514657842828 ) ) ;
#7643=FACE_OUTER_BOUND ( 'NONE', #8763, .T. ) ;
#7650=CARTESIAN_POINT ( 'NONE',  ( 49.28028498622276032, 34.52875999999999834, -25.68670502218146368 ) ) ;
#7653=CYLINDRICAL_SURFACE ( 'NONE', #13825, 1.190625000000000711 ) ;
#7657=LINE ( 'NONE', #19592, #7821 ) ;
#7658=ADVANCED_FACE ( 'NONE', ( #14449 ), #11119, .F. ) ;
#7672=CYLINDRICAL_SURFACE ( 'NONE', #13521, 0.7950199999999982836 ) ;
#7673=FACE_OUTER_BOUND ( 'NONE', #21179, .T. ) ;
#7674=CARTESIAN_POINT ( 'NONE',  ( 43.29176983217143260, 32.54502000000000095, 5.154088326438659884 ) ) ;
#7676=CIRCLE ( 'NONE', #2740, 0.5079999999999996740 ) ;
#7678=B_SPLINE_CURVE_WITH_KNOTS ( 'NONE', 3,
 ( #20188, #10038, #8365, #15138 ),
 .UNSPECIFIED., .F., .F.,
 ( 4, 4 ),
 ( -7.968845587668732479E-05, 0.0007517676470877217038 ),
 .UNSPECIFIED. ) ;
#7688=ORIENTED_EDGE ( 'NONE', *, *, #6976, .F. ) ;
#7690=CARTESIAN_POINT ( 'NONE',  ( 39.79795571586765845, -6.669711430507633487, -3.121712638490365510 ) ) ;
#7695=VERTEX_POINT ( 'NONE', #1163 ) ;
#7699=FACE_BOUND ( 'NONE', #7620, .T. ) ;
#7701=DIRECTION ( 'NONE',  ( -0.4987171968201928873, 0.000000000000000000, 0.8667647648559606566 ) ) ;
#7702=FACE_OUTER_BOUND ( 'NONE', #1940, .T. ) ;
#7713=ORIENTED_EDGE ( 'NONE', *, *, #16577, .F. ) ;
#7715=CARTESIAN_POINT ( 'NONE',  ( 52.27714366836601556, -6.669713112672388533, -17.51569705283379363 ) ) ;
#7720=DIRECTION ( 'NONE',  ( 0.000000000000000000, 1.000000000000000000, 0.000000000000000000 ) ) ;
#7721=DIRECTION ( 'NONE',  ( 0.000000000000000000, -1.000000000000000000, -0.000000000000000000 ) ) ;
#7724=ORIENTED_EDGE ( 'NONE', *, *, #18775, .T. ) ;
#7726=DIRECTION ( 'NONE',  ( 0.05085730733808139364, 0.000000000000000000, -0.9987059298363658577 ) ) ;
#7728=CARTESIAN_POINT ( 'NONE',  ( 53.69636427252483202, 38.88803500000000213, -18.48840734645144224 ) ) ;
#7745=DIRECTION ( 'NONE',  ( 0.000000000000000000, 1.000000000000000000, 0.000000000000000000 ) ) ;
#7746=VECTOR ( 'NONE', #20115, 1000.000000000000000 ) ;
#7748=EDGE_CURVE ( 'NONE', #3547, #3091, #13123, .T. ) ;
#7750=FACE_OUTER_BOUND ( 'NONE', #12553, .T. ) ;
#7770=AXIS2_PLACEMENT_3D ( 'NONE', #21488, #13012, #17971 ) ;
#7773=ADVANCED_FACE ( 'NONE', ( #13251 ), #13137, .T. ) ;
#7774=CIRCLE ( 'NONE', #20454, 30.16249999999998721 ) ;
#7779=CARTESIAN_POINT ( 'NONE',  ( 32.52436584422698473, 32.54502000000000095, 1.884807767196291284 ) ) ;
#7793=AXIS2_PLACEMENT_3D ( 'NONE', #6563, #13000, #7997 ) ;
#7795=DIRECTION ( 'NONE',  ( 0.9784543669157944601, 0.000000000000000000, 0.2064631973582987667 ) ) ;
#7814=DIRECTION ( 'NONE',  ( 0.7421532822901579785, 0.000000000000000000, -0.6702301885068630005 ) ) ;
#7819=CIRCLE ( 'NONE', #20503, 9.525000000000000355 ) ;
#7821=VECTOR ( 'NONE', #2904, 1000.000000000000000 ) ;
#7822=EDGE_CURVE ( 'NONE', #16730, #1384, #3063, .T. ) ;
#7833=CARTESIAN_POINT ( 'NONE',  ( 42.66304184606194383, 42.06303499999999929, -19.22597499813143784 ) ) ;
#7839=VERTEX_POINT ( 'NONE', #7922 ) ;
#7845=CIRCLE ( 'NONE', #11368, 0.5079999999999963434 ) ;
#7847=CARTESIAN_POINT ( 'NONE',  ( 39.16413618835606769, 32.54502000000000095, -24.45043885672975392 ) ) ;
#7855=AXIS2_PLACEMENT_3D ( 'NONE', #10190, #13985, #3788 ) ;
#7857=CARTESIAN_POINT ( 'NONE',  ( 52.91086381164393515, 0.000000000000000000, 3.812938856729753301 ) ) ;
#7858=CARTESIAN_POINT ( 'NONE',  ( 46.03750000000000142, 32.54502000000000095, -10.31874999999999964 ) ) ;
#7863=DIRECTION ( 'NONE',  ( -0.6702301885068632226, 0.000000000000000000, -0.7421532822901576454 ) ) ;
#7866=CARTESIAN_POINT ( 'NONE',  ( 45.99559936598748777, 32.54502000000000095, 5.449572532947073000 ) ) ;
#7867=AXIS2_PLACEMENT_3D ( 'NONE', #11001, #10791, #17536 ) ;
#7869=ORIENTED_EDGE ( 'NONE', *, *, #12821, .F. ) ;
#7874=VERTEX_POINT ( 'NONE', #18101 ) ;
#7878=CIRCLE ( 'NONE', #18114, 0.5079999999999995630 ) ;
#7887=CARTESIAN_POINT ( 'NONE',  ( 32.18388890846549799, 0.000000000000000000, 1.507793899792891468 ) ) ;
#7900=LINE ( 'NONE', #6345, #11702 ) ;
#7902=EDGE_CURVE ( 'NONE', #1582, #14783, #17707, .T. ) ;
#7905=ORIENTED_EDGE ( 'NONE', *, *, #9789, .T. ) ;
#7908=CIRCLE ( 'NONE', #20964, 0.5080000000000023386 ) ;
#7915=CARTESIAN_POINT ( 'NONE',  ( 38.24394060764427650, 39.20076311267237656, -4.842470972476202284 ) ) ;
#7917=VECTOR ( 'NONE', #7721, 1000.000000000000000 ) ;
#7922=CARTESIAN_POINT ( 'NONE',  ( 38.60701496492545459, 32.54502000000000095, -26.94161103631838472 ) ) ;
#7923=AXIS2_PLACEMENT_3D ( 'NONE', #16205, #9100, #602 ) ;
#7924=ORIENTED_EDGE ( 'NONE', *, *, #17072, .T. ) ;
#7925=ORIENTED_EDGE ( 'NONE', *, *, #19281, .F. ) ;
#7926=DIRECTION ( 'NONE',  ( -0.6702301885068652210, 0.000000000000000000, -0.7421532822901560911 ) ) ;
#7935=CIRCLE ( 'NONE', #11825, 0.7950199999999993938 ) ;
#7940=CARTESIAN_POINT ( 'NONE',  ( 52.49113927203449492, -6.356984999999999886, -16.14695822742181619 ) ) ;
#7945=VERTEX_POINT ( 'NONE', #8864 ) ;
#7950=CARTESIAN_POINT ( 'NONE',  ( 53.76119506325677122, 39.48900909932986281, -15.89313734090458397 ) ) ;
#7951=ORIENTED_EDGE ( 'NONE', *, *, #18149, .T. ) ;
#7955=CYLINDRICAL_SURFACE ( 'NONE', #18417, 30.16249999999999076 ) ;
#7957=ORIENTED_EDGE ( 'NONE', *, *, #8999, .T. ) ;
#7959=VERTEX_POINT ( 'NONE', #8451 ) ;
#7966=DIRECTION ( 'NONE',  ( 0.6496772031432432870, 0.000000000000000000, -0.7602101891687411683 ) ) ;
#7967=FACE_BOUND ( 'NONE', #21837, .T. ) ;
#7970=ORIENTED_EDGE ( 'NONE', *, *, #15268, .T. ) ;
#7972=DIRECTION ( 'NONE',  ( -0.9959941601142525691, 0.000000000000000000, -0.08941830359777946935 ) ) ;
#7976=DIRECTION ( 'NONE',  ( 0.05085730733808142834, 0.000000000000000000, -0.9987059298363657467 ) ) ;
#7981=ADVANCED_FACE ( 'NONE', ( #17277 ), #18924, .T. ) ;
#7984=CARTESIAN_POINT ( 'NONE',  ( 36.80301088673436283, -1.983739999999999837, -23.10021947667301134 ) ) ;
#7987=LINE ( 'NONE', #14863, #12527 ) ;
#7991=LINE ( 'NONE', #1463, #4712 ) ;
#7992=DIRECTION ( 'NONE',  ( 0.000000000000000000, 1.000000000000000000, -0.000000000000000000 ) ) ;
#7994=CARTESIAN_POINT ( 'NONE',  ( 52.94935177953276195, 40.07877905746412495, -16.57402588728236381 ) ) ;
#7997=DIRECTION ( 'NONE',  ( -0.7532174416907910786, 0.000000000000000000, -0.6577716059034319773 ) ) ;
#7998=VERTEX_POINT ( 'NONE', #3795 ) ;
#7999=CARTESIAN_POINT ( 'NONE',  ( 45.99559936598748777, 0.000000000000000000, 5.449572532947073000 ) ) ;
#8005=CARTESIAN_POINT ( 'NONE',  ( 52.98023334790573102, 37.69393439911831933, -16.84172433709920469 ) ) ;
#8019=CARTESIAN_POINT ( 'NONE',  ( 38.36548343274824902, 39.62000810270092188, -4.672696708993173687 ) ) ;
#8022=ADVANCED_FACE ( 'NONE', ( #10531 ), #20162, .T. ) ;
#8024=DIRECTION ( 'NONE',  ( 0.000000000000000000, -1.000000000000000000, -0.000000000000000000 ) ) ;
#8031=CARTESIAN_POINT ( 'NONE',  ( 50.52547294529469468, 38.88803500000000213, -18.64987929725020521 ) ) ;
#8036=ORIENTED_EDGE ( 'NONE', *, *, #13314, .F. ) ;
#8041=CARTESIAN_POINT ( 'NONE',  ( 50.62387473582167274, 32.54502000000000095, -28.41576006634952734 ) ) ;
#8042=EDGE_CURVE ( 'NONE', #18076, #12952, #12423, .T. ) ;
#8043=CARTESIAN_POINT ( 'NONE',  ( 44.27024749654656688, 38.88803500000000213, -8.722764363618033201 ) ) ;
#8050=CARTESIAN_POINT ( 'NONE',  ( 30.97944403357121956, 0.000000000000000000, -8.103300075789407586 ) ) ;
#8053=DIRECTION ( 'NONE',  ( 0.000000000000000000, 1.000000000000000000, 0.000000000000000000 ) ) ;
#8058=CYLINDRICAL_SURFACE ( 'NONE', #17913, 1.190624999999999822 ) ;
#8060=ORIENTED_EDGE ( 'NONE', *, *, #13327, .F. ) ;
#8061=ORIENTED_EDGE ( 'NONE', *, *, #9791, .T. ) ;
#8062=CARTESIAN_POINT ( 'NONE',  ( 53.25483508941461963, 34.52875999999999834, -5.879799058943532941 ) ) ;
#8067=CYLINDRICAL_SURFACE ( 'NONE', #15545, 1.190624999999999822 ) ;
#8075=DIRECTION ( 'NONE',  ( 0.000000000000000000, -1.000000000000000000, 0.000000000000000000 ) ) ;
#8080=DIRECTION ( 'NONE',  ( -0.7421532822901579785, 0.000000000000000000, 0.6702301885068630005 ) ) ;
#8082=EDGE_LOOP ( 'NONE', ( #2656, #19743, #13384, #2849, #19189, #4840 ) ) ;
#8086=AXIS2_PLACEMENT_3D ( 'NONE', #7984, #4467, #1247 ) ;
#8088=DIRECTION ( 'NONE',  ( 0.1060008583745224581, 0.000000000000000000, 0.9943660382494288186 ) ) ;
#8098=CARTESIAN_POINT ( 'NONE',  ( 40.21953902438700368, -6.356984999999999886, -3.460331122294329820 ) ) ;
#8101=EDGE_CURVE ( 'NONE', #13851, #13712, #2884, .T. ) ;
#8108=CARTESIAN_POINT ( 'NONE',  ( 46.03750000000000142, 42.06303499999999929, -10.31874999999999964 ) ) ;
#8109=VERTEX_POINT ( 'NONE', #16918 ) ;
#8112=ORIENTED_EDGE ( 'NONE', *, *, #52, .T. ) ;
#8118=VERTEX_POINT ( 'NONE', #19909 ) ;
#8128=CIRCLE ( 'NONE', #4606, 0.5080000000000002292 ) ;
#8133=VERTEX_POINT ( 'NONE', #3113 ) ;
#8136=LINE ( 'NONE', #6372, #6033 ) ;
#8140=AXIS2_PLACEMENT_3D ( 'NONE', #1217, #21766, #18239 ) ;
#8147=VECTOR ( 'NONE', #20688, 1000.000000000000000 ) ;
#8158=AXIS2_PLACEMENT_3D ( 'NONE', #18191, #11332, #11547 ) ;
#8167=ORIENTED_EDGE ( 'NONE', *, *, #18725, .F. ) ;
#8173=CIRCLE ( 'NONE', #8513, 30.16249999999999432 ) ;
#8174=EDGE_CURVE ( 'NONE', #13027, #12952, #8956, .T. ) ;
#8177=CIRCLE ( 'NONE', #9575, 0.5080000000000000071 ) ;
#8179=CIRCLE ( 'NONE', #763, 30.16249999999999432 ) ;
#8185=CARTESIAN_POINT ( 'NONE',  ( 38.82016491058538321, 42.06303499999999929, -14.75770094105646812 ) ) ;
#8186=ORIENTED_EDGE ( 'NONE', *, *, #4296, .F. ) ;
#8189=CYLINDRICAL_SURFACE ( 'NONE', #18416, 1.190625000000000711 ) ;
#8192=VERTEX_POINT ( 'NONE', #18789 ) ;
#8195=DIRECTION ( 'NONE',  ( -0.6702301885068632226, 0.000000000000000000, -0.7421532822901576454 ) ) ;
#8198=AXIS2_PLACEMENT_3D ( 'NONE', #3957, #18758, #299 ) ;
#8205=ADVANCED_FACE ( 'NONE', ( #13965 ), #10663, .T. ) ;
#8213=AXIS2_PLACEMENT_3D ( 'NONE', #19302, #19196, #19406 ) ;
#8214=CARTESIAN_POINT ( 'NONE',  ( 61.65536943582333151, 34.52875999999999834, -11.98363747855214712 ) ) ;
#8221=CARTESIAN_POINT ( 'NONE',  ( 32.42378190387104553, -1.983739999999999837, -18.15178106273469183 ) ) ;
#8223=ORIENTED_EDGE ( 'NONE', *, *, #3537, .F. ) ;
#8225=LINE ( 'NONE', #20138, #4231 ) ;
#8227=DIRECTION ( 'NONE',  ( 0.000000000000000000, 1.000000000000000000, 0.000000000000000000 ) ) ;
#8232=EDGE_CURVE ( 'NONE', #13313, #10898, #9588, .T. ) ;
#8235=DIRECTION ( 'NONE',  ( 0.000000000000000000, -1.000000000000000000, -0.000000000000000000 ) ) ;
#8239=CIRCLE ( 'NONE', #10007, 1.190624999999999378 ) ;
#8243=DIRECTION ( 'NONE',  ( -0.6702301885068628895, 0.000000000000000000, -0.7421532822901579785 ) ) ;
#8244=AXIS2_PLACEMENT_3D ( 'NONE', #9402, #900, #13365 ) ;
#8251=DIRECTION ( 'NONE',  ( 0.3542738219355867080, 0.000000000000000000, 0.9351417320872553729 ) ) ;
#8254=ORIENTED_EDGE ( 'NONE', *, *, #9616, .F. ) ;
#8256=CIRCLE ( 'NONE', #2257, 9.525000000000002132 ) ;
#8257=ORIENTED_EDGE ( 'NONE', *, *, #12938, .T. ) ;
#8259=VERTEX_POINT ( 'NONE', #9059 ) ;
#8261=ORIENTED_EDGE ( 'NONE', *, *, #21034, .F. ) ;
#8265=AXIS2_PLACEMENT_3D ( 'NONE', #21591, #19928, #4472 ) ;
#8266=CARTESIAN_POINT ( 'NONE',  ( 56.91751438644678984, -1.983739999999999837, -20.96198986413465448 ) ) ;
#8270=DIRECTION ( 'NONE',  ( 0.000000000000000000, -1.000000000000000000, -0.000000000000000000 ) ) ;
#8273=EDGE_CURVE ( 'NONE', #13394, #14493, #5194, .T. ) ;
#8276=ORIENTED_EDGE ( 'NONE', *, *, #16436, .T. ) ;
#8278=DIRECTION ( 'NONE',  ( 0.000000000000000000, 1.000000000000000000, -0.000000000000000000 ) ) ;
#8285=EDGE_CURVE ( 'NONE', #1068, #20066, #8177, .T. ) ;
#8296=DIRECTION ( 'NONE',  ( 0.000000000000000000, 1.000000000000000000, 0.000000000000000000 ) ) ;
#8300=EDGE_LOOP ( 'NONE', ( #10554, #20666, #4501, #4410 ) ) ;
#8304=VERTEX_POINT ( 'NONE', #11947 ) ;
#8306=CARTESIAN_POINT ( 'NONE',  ( 32.96560389001691505, 34.52875999999999834, -17.84002872454335886 ) ) ;
#8307=DIRECTION ( 'NONE',  ( -0.6702301885068634446, 0.000000000000000000, -0.7421532822901576454 ) ) ;
#8312=CIRCLE ( 'NONE', #17144, 0.5080000000000013394 ) ;
#8318=DIRECTION ( 'NONE',  ( 0.9943660382494290406, 0.000000000000000000, -0.1060008583745199739 ) ) ;
#8325=EDGE_CURVE ( 'NONE', #1509, #5503, #4303, .T. ) ;
#8326=VERTEX_POINT ( 'NONE', #225 ) ;
#8357=ORIENTED_EDGE ( 'NONE', *, *, #11423, .T. ) ;
#8359=ORIENTED_EDGE ( 'NONE', *, *, #20820, .T. ) ;
#8362=ORIENTED_EDGE ( 'NONE', *, *, #10292, .T. ) ;
#8363=B_SPLINE_CURVE_WITH_KNOTS ( 'NONE', 3,
 ( #15995, #2593, #7570, #929, #14331, #12660, #21151, #19386, #12776, #19499, #4362, #3032 ),
 .UNSPECIFIED., .F., .F.,
 ( 4, 2, 2, 2, 2, 4 ),
 ( 0.001233369978144762671, 0.001719813969628884937, 0.001963035965370948238, 0.002206257961113011756, 0.002692701952597139660, 0.003179145944081267997 ),
 .UNSPECIFIED. ) ;
#8365=CARTESIAN_POINT ( 'NONE',  ( 39.18468883297455818, 40.07906110073898276, -4.105455453847051572 ) ) ;
#8370=DIRECTION ( 'NONE',  ( -0.000000000000000000, -1.000000000000000000, 0.000000000000000000 ) ) ;
#8373=VERTEX_POINT ( 'NONE', #11269 ) ;
#8377=VERTEX_POINT ( 'NONE', #9496 ) ;
#8380=ORIENTED_EDGE ( 'NONE', *, *, #3975, .T. ) ;
#8383=FACE_OUTER_BOUND ( 'NONE', #3262, .T. ) ;
#8388=ADVANCED_FACE ( 'NONE', ( #19565, #20887 ), #4204, .T. ) ;
#8394=CARTESIAN_POINT ( 'NONE',  ( 53.00094895929537842, -7.547610000000004149, -16.81958146583652791 ) ) ;
#8406=EDGE_CURVE ( 'NONE', #4430, #18428, #11720, .T. ) ;
#8408=CARTESIAN_POINT ( 'NONE',  ( 34.72145145287101542, -1.983739999999999837, 0.5851394578805096947 ) ) ;
#8410=DIRECTION ( 'NONE',  ( -0.9987059298363657467, 0.000000000000000000, -0.05085730733808445370 ) ) ;
#8411=VECTOR ( 'NONE', #6675, 1000.000000000000000 ) ;
#8415=CARTESIAN_POINT ( 'NONE',  ( 53.28913209022548614, -6.356984999999999886, -15.26333197569509714 ) ) ;
#8418=FACE_OUTER_BOUND ( 'NONE', #20714, .T. ) ;
#8420=FACE_BOUND ( 'NONE', #20924, .T. ) ;
#8422=DIRECTION ( 'NONE',  ( 0.7421532822901579785, 0.000000000000000000, -0.6702301885068630005 ) ) ;
#8430=DIRECTION ( 'NONE',  ( -0.6702301885068630005, 0.000000000000000000, -0.7421532822901579785 ) ) ;
#8436=EDGE_CURVE ( 'NONE', #3189, #180, #756, .T. ) ;
#8438=EDGE_CURVE ( 'NONE', #13139, #18598, #13141, .T. ) ;
#8451=CARTESIAN_POINT ( 'NONE',  ( 35.15748561355322011, 34.52875999999999834, 0.3244898641346534163 ) ) ;
#8459=ORIENTED_EDGE ( 'NONE', *, *, #8673, .F. ) ;
#8465=LINE ( 'NONE', #21852, #9696 ) ;
#8466=EDGE_LOOP ( 'NONE', ( #18648, #9569, #2189 ) ) ;
#8467=APPLICATION_CONTEXT ( 'automotive_design' ) ;
#8469=AXIS2_PLACEMENT_3D ( 'NONE', #9078, #17718, #15853 ) ;
#8471=CARTESIAN_POINT ( 'NONE',  ( 39.58386072796507449, 40.07865999999999929, -4.490541772578644064 ) ) ;
#8472=CYLINDRICAL_SURFACE ( 'NONE', #21021, 0.5079999999999984528 ) ;
#8474=ORIENTED_EDGE ( 'NONE', *, *, #2395, .F. ) ;
#8475=CARTESIAN_POINT ( 'NONE',  ( 59.65121809612895731, 34.52875999999999834, -2.485718937265306572 ) ) ;
#8479=CARTESIAN_POINT ( 'NONE',  ( 59.65121809612895731, 32.54502000000000095, -2.485718937265306572 ) ) ;
#8481=VERTEX_POINT ( 'NONE', #12614 ) ;
#8482=ORIENTED_EDGE ( 'NONE', *, *, #3741, .F. ) ;
#8499=LINE ( 'NONE', #10394, #11211 ) ;
#8500=ADVANCED_FACE ( 'NONE', ( #15947 ), #7955, .T. ) ;
#8501=ORIENTED_EDGE ( 'NONE', *, *, #8938, .T. ) ;
#8504=DIRECTION ( 'NONE',  ( -0.6702301885068632226, 0.000000000000000000, -0.7421532822901576454 ) ) ;
#8510=CARTESIAN_POINT ( 'NONE',  ( 39.42154620619601957, -6.356984999999999886, -4.343957374021048423 ) ) ;
#8512=ORIENTED_EDGE ( 'NONE', *, *, #15233, .T. ) ;
#8513=AXIS2_PLACEMENT_3D ( 'NONE', #17170, #15653, #20925 ) ;
#8514=ORIENTED_EDGE ( 'NONE', *, *, #21801, .T. ) ;
#8532=ORIENTED_EDGE ( 'NONE', *, *, #16140, .T. ) ;
#8533=LINE ( 'NONE', #10196, #11395 ) ;
#8543=CARTESIAN_POINT ( 'NONE',  ( 32.42378190387104553, 0.000000000000000000, -18.15178106273469183 ) ) ;
#8550=EDGE_CURVE ( 'NONE', #7171, #18389, #5720, .T. ) ;
#8553=VERTEX_POINT ( 'NONE', #3855 ) ;
#8554=VECTOR ( 'NONE', #9127, 1000.000000000000114 ) ;
#8573=EDGE_LOOP ( 'NONE', ( #8112, #1538, #15065, #18880 ) ) ;
#8577=ADVANCED_FACE ( 'NONE', ( #12368 ), #20524, .F. ) ;
#8579=AXIS2_PLACEMENT_3D ( 'NONE', #4725, #9463, #17661 ) ;
#8586=CARTESIAN_POINT ( 'NONE',  ( 42.35466991749225940, 32.54502000000000095, -17.94967221382040279 ) ) ;
#8588=FACE_BOUND ( 'NONE', #14386, .T. ) ;
#8590=DIRECTION ( 'NONE',  ( 0.000000000000000000, 1.000000000000000000, 0.000000000000000000 ) ) ;
#8611=CIRCLE ( 'NONE', #17095, 30.16250000000000497 ) ;
#8616=EDGE_LOOP ( 'NONE', ( #11845, #14281, #15393, #3314 ) ) ;
#8619=CARTESIAN_POINT ( 'NONE',  ( 37.29356535768673098, -6.356984999999999886, -6.700294045292300105 ) ) ;
#8622=CARTESIAN_POINT ( 'NONE',  ( 42.35466991749225940, 32.54502000000000095, -17.94967221382040279 ) ) ;
#8624=ADVANCED_FACE ( 'NONE', ( #6843 ), #18879, .F. ) ;
#8626=DIRECTION ( 'NONE',  ( 0.000000000000000000, -1.000000000000000000, -0.000000000000000000 ) ) ;
#8646=CARTESIAN_POINT ( 'NONE',  ( 39.07078961959606289, 0.000000000000000000, -27.14892015257980162 ) ) ;
#8660=LINE ( 'NONE', #11988, #16411 ) ;
#8662=ORIENTED_EDGE ( 'NONE', *, *, #68, .F. ) ;
#8664=EDGE_CURVE ( 'NONE', #1990, #13930, #424, .T. ) ;
#8672=ORIENTED_EDGE ( 'NONE', *, *, #872, .F. ) ;
#8673=EDGE_CURVE ( 'NONE', #21216, #4173, #10709, .T. ) ;
#8687=DIRECTION ( 'NONE',  ( 0.000000000000000000, -1.000000000000000000, 0.000000000000000000 ) ) ;
#8688=CARTESIAN_POINT ( 'NONE',  ( 32.04318496342826705, -6.356984999999999886, -2.596378499983996946 ) ) ;
#8695=FACE_OUTER_BOUND ( 'NONE', #11568, .T. ) ;
#8697=CARTESIAN_POINT ( 'NONE',  ( 52.44708915697334106, 32.54502000000000095, 4.020247972991190188 ) ) ;
#8704=ORIENTED_EDGE ( 'NONE', *, *, #12768, .T. ) ;
#8706=ADVANCED_FACE ( 'NONE', ( #12259 ), #5273, .F. ) ;
#8707=ORIENTED_EDGE ( 'NONE', *, *, #18123, .F. ) ;
#8710=ORIENTED_EDGE ( 'NONE', *, *, #13409, .T. ) ;
#8715=EDGE_CURVE ( 'NONE', #19210, #15662, #14044, .T. ) ;
#8718=CARTESIAN_POINT ( 'NONE',  ( 47.80475250345343596, 37.69740999999999786, -11.91473563638196786 ) ) ;
#8721=AXIS2_PLACEMENT_3D ( 'NONE', #13247, #6587, #8243 ) ;
#8724=CARTESIAN_POINT ( 'NONE',  ( 39.27728671717661513, 34.52875999999999834, -23.95520057284206672 ) ) ;
#8739=EDGE_CURVE ( 'NONE', #1050, #19416, #745, .T. ) ;
#8741=DIRECTION ( 'NONE',  ( 0.6702301885068632226, 0.000000000000000000, 0.7421532822901576454 ) ) ;
#8745=DIRECTION ( 'NONE',  ( 0.000000000000000000, 1.000000000000000000, 0.000000000000000000 ) ) ;
#8748=DIRECTION ( 'NONE',  ( 0.6702301885068630005, 0.000000000000000000, 0.7421532822901579785 ) ) ;
#8750=CYLINDRICAL_SURFACE ( 'NONE', #20506, 0.5079999999999995630 ) ;
#8755=DIRECTION ( 'NONE',  ( 0.000000000000000000, 1.000000000000000000, 0.000000000000000000 ) ) ;
#8760=CARTESIAN_POINT ( 'NONE',  ( 53.14266576735293768, -5.167590446840315543, -16.66242751532468702 ) ) ;
#8761=EDGE_CURVE ( 'NONE', #17518, #5857, #21556, .T. ) ;
#8763=EDGE_LOOP ( 'NONE', ( #2572, #21674, #11778, #19942, #12920 ) ) ;
#8768=CARTESIAN_POINT ( 'NONE',  ( 46.07940063401251507, 32.54502000000000095, -26.08707253294707229 ) ) ;
#8769=VECTOR ( 'NONE', #5788, 1000.000000000000114 ) ;
#8771=UNCERTAINTY_MEASURE_WITH_UNIT (LENGTH_MEASURE( 1.000000000000000082E-05 ), #19730, 'distance_accuracy_value', 'NONE');
#8787=AXIS2_PLACEMENT_3D ( 'NONE', #16613, #11515, #21461 ) ;
#8789=DIRECTION ( 'NONE',  ( -0.8667647648559581031, 0.000000000000000000, -0.4987171968201974948 ) ) ;
#8791=ADVANCED_FACE ( 'NONE', ( #5730 ), #11242, .F. ) ;
#8792=CARTESIAN_POINT ( 'NONE',  ( 34.38097451710952868, 34.52875999999999834, 0.2081255904771098786 ) ) ;
#8804=ORIENTED_EDGE ( 'NONE', *, *, #12135, .T. ) ;
#8813=EDGE_LOOP ( 'NONE', ( #16256, #9089, #8036, #10255 ) ) ;
#8814=AXIS2_PLACEMENT_3D ( 'NONE', #13231, #19941, #4814 ) ;
#8818=ORIENTED_EDGE ( 'NONE', *, *, #6643, .T. ) ;
#8824=CARTESIAN_POINT ( 'NONE',  ( 38.84151346225866774, -7.551139666418512419, -4.076215976391670992 ) ) ;
#8829=CIRCLE ( 'NONE', #3197, 30.16249999999998721 ) ;
#8830=VERTEX_POINT ( 'NONE', #2735 ) ;
#8832=DIRECTION ( 'NONE',  ( -0.6702301885068628895, 0.000000000000000000, -0.7421532822901579785 ) ) ;
#8851=DIRECTION ( 'NONE',  ( -0.9987059298363656357, 0.000000000000000000, -0.05085730733808393328 ) ) ;
#8854=CARTESIAN_POINT ( 'NONE',  ( 32.17043356788648367, 37.11476346399999926, -17.71146456218788146 ) ) ;
#8857=CARTESIAN_POINT ( 'NONE',  ( 38.60701496492545459, -1.983739999999999837, -26.94161103631838472 ) ) ;
#8864=CARTESIAN_POINT ( 'NONE',  ( 32.55306802826559220, 34.52875999999999834, -17.37731658638881527 ) ) ;
#8867=DIRECTION ( 'NONE',  ( 0.000000000000000000, 1.000000000000000000, 0.000000000000000000 ) ) ;
#8869=CIRCLE ( 'NONE', #20521, 1.984375000000000000 ) ;
#8894=CIRCLE ( 'NONE', #430, 0.7950199999999982836 ) ;
#8902=EDGE_LOOP ( 'NONE', ( #16017, #5040, #4435, #8380 ) ) ;
#8905=CYLINDRICAL_SURFACE ( 'NONE', #11252, 0.5079999999999996740 ) ;
#8908=DIRECTION ( 'NONE',  ( -0.9987059298363656357, 0.000000000000000000, -0.05085730733808393328 ) ) ;
#8911=LINE ( 'NONE', #2399, #21631 ) ;
#8914=DIRECTION ( 'NONE',  ( 0.000000000000000000, 1.000000000000000000, 0.000000000000000000 ) ) ;
#8918=VERTEX_POINT ( 'NONE', #4293 ) ;
#8925=ORIENTED_EDGE ( 'NONE', *, *, #14569, .F. ) ;
#8930=VERTEX_POINT ( 'NONE', #6045 ) ;
#8934=ORIENTED_EDGE ( 'NONE', *, *, #21176, .T. ) ;
#8938=EDGE_CURVE ( 'NONE', #4294, #2096, #7090, .T. ) ;
#8940=AXIS2_PLACEMENT_3D ( 'NONE', #4499, #4607, #12689 ) ;
#8941=CARTESIAN_POINT ( 'NONE',  ( 38.20353551528305047, -6.675755166547726382, -4.900394175645134354 ) ) ;
#8942=CARTESIAN_POINT ( 'NONE',  ( 59.89111109153450485, 0.000000000000000000, -22.14529389979288965 ) ) ;
#8943=DIRECTION ( 'NONE',  ( -0.05085730733808459941, 0.000000000000000000, 0.9987059298363656357 ) ) ;
#8946=ORIENTED_EDGE ( 'NONE', *, *, #9301, .T. ) ;
#8951=EDGE_CURVE ( 'NONE', #18019, #12607, #14879, .T. ) ;
#8956=LINE ( 'NONE', #12177, #15623 ) ;
#8969=CARTESIAN_POINT ( 'NONE',  ( 39.58386072796550081, 38.88803500000000213, -4.490541772578183100 ) ) ;
#8974=DIRECTION ( 'NONE',  ( 0.000000000000000000, 1.000000000000000000, 0.000000000000000000 ) ) ;
#8977=AXIS2_PLACEMENT_3D ( 'NONE', #20711, #2481, #5567 ) ;
#8978=DIRECTION ( 'NONE',  ( -0.9129422336036127072, 0.000000000000000000, 0.4080888115384278536 ) ) ;
#8981=VERTEX_POINT ( 'NONE', #16562 ) ;
#8985=AXIS2_PLACEMENT_3D ( 'NONE', #13124, #8235, #19837 ) ;
#8986=ORIENTED_EDGE ( 'NONE', *, *, #758, .T. ) ;
#8999=EDGE_CURVE ( 'NONE', #1735, #7286, #20784, .T. ) ;
#9006=AXIS2_PLACEMENT_3D ( 'NONE', #17959, #6007, #17856 ) ;
#9007=EDGE_LOOP ( 'NONE', ( #11475, #20386, #14705 ) ) ;
#9009=CARTESIAN_POINT ( 'NONE',  ( 53.10651001381376091, -5.166360000000002728, -16.70269254552787075 ) ) ;
#9017=LINE ( 'NONE', #17315, #13566 ) ;
#9020=CARTESIAN_POINT ( 'NONE',  ( 30.41963056417667488, 0.000000000000000000, -8.653862521447852174 ) ) ;
#9023=EDGE_CURVE ( 'NONE', #3908, #6031, #8136, .T. ) ;
#9035=VERTEX_POINT ( 'NONE', #18108 ) ;
#9039=ORIENTED_EDGE ( 'NONE', *, *, #21034, .T. ) ;
#9044=DIRECTION ( 'NONE',  ( 0.000000000000000000, -1.000000000000000000, -0.000000000000000000 ) ) ;
#9053=DIRECTION ( 'NONE',  ( -0.9129422336036122632, 0.000000000000000000, 0.4080888115384288528 ) ) ;
#9057=AXIS2_PLACEMENT_3D ( 'NONE', #4370, #4806, #16211 ) ;
#9059=CARTESIAN_POINT ( 'NONE',  ( 37.19264538843808765, -6.356984999999999886, -4.718486965773546871 ) ) ;
#9061=ORIENTED_EDGE ( 'NONE', *, *, #10717, .F. ) ;
#9066=DIRECTION ( 'NONE',  ( 0.000000000000000000, -1.000000000000000000, -0.000000000000000000 ) ) ;
#9069=DIRECTION ( 'NONE',  ( -0.9987059298363656357, 0.000000000000000000, -0.05085730733808393328 ) ) ;
#9070=ADVANCED_FACE ( 'NONE', ( #13144 ), #1089, .T. ) ;
#9071=VECTOR ( 'NONE', #16062, 1000.000000000000114 ) ;
#9073=EDGE_CURVE ( 'NONE', #19208, #15022, #3168, .T. ) ;
#9078=CARTESIAN_POINT ( 'NONE',  ( 32.17043356788648367, -1.983739999999999837, -17.71146456218788146 ) ) ;
#9089=ORIENTED_EDGE ( 'NONE', *, *, #18579, .F. ) ;
#9094=ORIENTED_EDGE ( 'NONE', *, *, #2742, .T. ) ;
#9099=VECTOR ( 'NONE', #991, 1000.000000000000000 ) ;
#9100=DIRECTION ( 'NONE',  ( 0.000000000000000000, 1.000000000000000000, 0.000000000000000000 ) ) ;
#9107=CARTESIAN_POINT ( 'NONE',  ( 27.40895291499714403, 0.000000000000000000, -9.088367920799473865 ) ) ;
#9108=VERTEX_POINT ( 'NONE', #11899 ) ;
#9116=EDGE_CURVE ( 'NONE', #17778, #21489, #15453, .T. ) ;
#9119=CARTESIAN_POINT ( 'NONE',  ( 38.23013820809905638, 109.3223030719999969, -14.22485453658974031 ) ) ;
#9127=DIRECTION ( 'NONE',  ( -0.7421532822901579785, 0.000000000000000000, 0.6702301885068628895 ) ) ;
#9133=LINE ( 'NONE', #18973, #21304 ) ;
#9136=ORIENTED_EDGE ( 'NONE', *, *, #19670, .F. ) ;
#9139=ORIENTED_EDGE ( 'NONE', *, *, #620, .F. ) ;
#9141=EDGE_CURVE ( 'NONE', #10543, #3115, #3557, .T. ) ;
#9144=ORIENTED_EDGE ( 'NONE', *, *, #6855, .T. ) ;
#9154=ORIENTED_EDGE ( 'NONE', *, *, #5218, .T. ) ;
#9165=EDGE_LOOP ( 'NONE', ( #1511, #8167, #11920, #20502 ) ) ;
#9167=EDGE_CURVE ( 'NONE', #18470, #18734, #6736, .T. ) ;
#9171=CYLINDRICAL_SURFACE ( 'NONE', #17957, 0.5079999999999984528 ) ;
#9181=DIRECTION ( 'NONE',  ( -0.6702301885068652210, 0.000000000000000000, -0.7421532822901560911 ) ) ;
#9193=CARTESIAN_POINT ( 'NONE',  ( 57.69402548289047417, -1.983739999999999837, -20.84562559047711261 ) ) ;
#9195=CIRCLE ( 'NONE', #12032, 0.7950199999999993938 ) ;
#9211=AXIS2_PLACEMENT_3D ( 'NONE', #20251, #18711, #3370 ) ;
#9216=ORIENTED_EDGE ( 'NONE', *, *, #19248, .T. ) ;
#9220=ORIENTED_EDGE ( 'NONE', *, *, #8664, .F. ) ;
#9239=CARTESIAN_POINT ( 'NONE',  ( 59.55063415577301811, 0.000000000000000000, -22.52230776719629191 ) ) ;
#9243=ORIENTED_EDGE ( 'NONE', *, *, #6025, .F. ) ;
#9248=DIRECTION ( 'NONE',  ( -0.6702301885068628895, 0.000000000000000000, -0.7421532822901579785 ) ) ;
#9255=EDGE_LOOP ( 'NONE', ( #19620, #17222, #10590, #19665 ) ) ;
#9258=VECTOR ( 'NONE', #5824, 1000.000000000000114 ) ;
#9260=AXIS2_PLACEMENT_3D ( 'NONE', #1357, #11213, #19933 ) ;
#9261=AXIS2_PLACEMENT_3D ( 'NONE', #7728, #16151, #6067 ) ;
#9263=EDGE_CURVE ( 'NONE', #21520, #3969, #3719, .T. ) ;
#9265=DIRECTION ( 'NONE',  ( 0.000000000000000000, 1.000000000000000000, 0.000000000000000000 ) ) ;
#9269=ADVANCED_FACE ( 'NONE', ( #2494 ), #12719, .T. ) ;
#9274=CARTESIAN_POINT ( 'NONE',  ( 30.24348838687780727, -1.983739999999999837, -20.27293523655082552 ) ) ;
#9275=AXIS2_PLACEMENT_3D ( 'NONE', #18544, #18440, #13476 ) ;
#9283=EDGE_LOOP ( 'NONE', ( #14550, #21284, #6368, #16645 ) ) ;
#9284=DIRECTION ( 'NONE',  ( 0.2227372614606430989, 0.000000000000000000, 0.9748785115885020280 ) ) ;
#9286=VECTOR ( 'NONE', #19925, 1000.000000000000000 ) ;
#9288=LINE ( 'NONE', #5531, #284 ) ;
#9296=CARTESIAN_POINT ( 'NONE',  ( 34.72145145287101542, 0.000000000000000000, 0.5851394578805096947 ) ) ;
#9297=CARTESIAN_POINT ( 'NONE',  ( 49.41195815393805901, 34.52875999999999834, -1.411525001868561224 ) ) ;
#9301=EDGE_CURVE ( 'NONE', #18266, #10543, #12339, .T. ) ;
#9302=CARTESIAN_POINT ( 'NONE',  ( 39.37900608539015224, 37.69740999999999786, -4.303192893338801284 ) ) ;
#9306=ORIENTED_EDGE ( 'NONE', *, *, #21801, .F. ) ;
#9307=CARTESIAN_POINT ( 'NONE',  ( 30.25543876212147509, -1.983739999999999837, -19.39939755251907272 ) ) ;
#9309=ORIENTED_EDGE ( 'NONE', *, *, #4072, .F. ) ;
#9310=VECTOR ( 'NONE', #2562, 1000.000000000000000 ) ;
#9319=CARTESIAN_POINT ( 'NONE',  ( 32.17043356788648367, 0.000000000000000000, -17.71146456218788146 ) ) ;
#9332=ORIENTED_EDGE ( 'NONE', *, *, #16549, .F. ) ;
#9333=AXIS2_PLACEMENT_3D ( 'NONE', #3584, #3376, #5129 ) ;
#9334=CYLINDRICAL_SURFACE ( 'NONE', #4223, 0.5080000000000022276 ) ;
#9338=CARTESIAN_POINT ( 'NONE',  ( 32.52436584422698473, 34.52875999999999834, 1.884807767196291284 ) ) ;
#9341=AXIS2_PLACEMENT_3D ( 'NONE', #2426, #4191, #17242 ) ;
#9349=DIRECTION ( 'NONE',  ( 0.000000000000000000, -1.000000000000000000, -0.000000000000000000 ) ) ;
#9357=CARTESIAN_POINT ( 'NONE',  ( 37.51913901087312553, -1.983739999999999837, -14.58057485080488114 ) ) ;
#9358=DIRECTION ( 'NONE',  ( -0.2064631973582987667, 0.000000000000000000, 0.9784543669157944601 ) ) ;
#9361=ORIENTED_EDGE ( 'NONE', *, *, #10075, .T. ) ;
#9367=EDGE_LOOP ( 'NONE', ( #21293, #19100, #4094, #8818 ) ) ;
#9370=VECTOR ( 'NONE', #11317, 1000.000000000000000 ) ;
#9379=ORIENTED_EDGE ( 'NONE', *, *, #1244, .F. ) ;
#9381=CARTESIAN_POINT ( 'NONE',  ( 54.78059207134182884, -6.356984999999999886, -16.96151288338074181 ) ) ;
#9383=FACE_OUTER_BOUND ( 'NONE', #2870, .T. ) ;
#9384=DIRECTION ( 'NONE',  ( 0.000000000000000000, 1.000000000000000000, 0.000000000000000000 ) ) ;
#9385=ADVANCED_FACE ( 'NONE', ( #5700 ), #16008, .T. ) ;
#9386=EDGE_LOOP ( 'NONE', ( #15707, #21873, #9603, #5985 ) ) ;
#9387=VERTEX_POINT ( 'NONE', #17432 ) ;
#9392=VERTEX_POINT ( 'NONE', #4049 ) ;
#9393=VERTEX_POINT ( 'NONE', #837 ) ;
#9399=EDGE_CURVE ( 'NONE', #19416, #1021, #1046, .T. ) ;
#9402=CARTESIAN_POINT ( 'NONE',  ( 61.04701390398659555, -1.983739999999999837, -15.15157976445104993 ) ) ;
#9406=CARTESIAN_POINT ( 'NONE',  ( 49.13030338002142372, 32.54502000000000095, -2.154981381712871791 ) ) ;
#9410=CARTESIAN_POINT ( 'NONE',  ( 39.18461504901784309, 37.69700956874092412, -4.105368993849036308 ) ) ;
#9412=CARTESIAN_POINT ( 'NONE',  ( 61.02111788801703085, 32.54502000000000095, -5.406220493519755088 ) ) ;
#9415=ORIENTED_EDGE ( 'NONE', *, *, #14997, .T. ) ;
#9428=CARTESIAN_POINT ( 'NONE',  ( 52.65345379380355695, 40.07865999999999929, -16.29354262597941982 ) ) ;
#9432=LINE ( 'NONE', #21149, #16024 ) ;
#9436=DIRECTION ( 'NONE',  ( -0.9987059298363656357, -0.000000000000000000, -0.05085730733808393328 ) ) ;
#9437=AXIS2_PLACEMENT_3D ( 'NONE', #5160, #17212, #7164 ) ;
#9439=CARTESIAN_POINT ( 'NONE',  ( 50.29383871662588490, 0.000000000000000000, -28.02957329025317179 ) ) ;
#9440=DIRECTION ( 'NONE',  ( -0.000000000000000000, -1.000000000000000000, 0.000000000000000000 ) ) ;
#9451=CARTESIAN_POINT ( 'NONE',  ( 39.07267844585335581, -7.547610000000000596, -3.819438423585947540 ) ) ;
#9461=CARTESIAN_POINT ( 'NONE',  ( 46.03750000000000142, 42.06303499999999929, -10.31874999999999964 ) ) ;
#9463=DIRECTION ( 'NONE',  ( 0.7421532822901579785, 0.000000000000000000, -0.6702301885068630005 ) ) ;
#9468=VECTOR ( 'NONE', #21792, 1000.000000000000000 ) ;
#9474=ORIENTED_EDGE ( 'NONE', *, *, #19924, .T. ) ;
#9481=CARTESIAN_POINT ( 'NONE',  ( 39.00487391864218267, 37.69864044684034354, -3.894748490052650780 ) ) ;
#9483=DIRECTION ( 'NONE',  ( 0.000000000000000000, -1.000000000000000000, -0.000000000000000000 ) ) ;
#9488=CARTESIAN_POINT ( 'NONE',  ( 53.00421038040393995, -4.569743463999999200, 6.511420152579801446 ) ) ;
#9489=DIRECTION ( 'NONE',  ( 0.000000000000000000, 1.000000000000000000, 0.000000000000000000 ) ) ;
#9490=ADVANCED_FACE ( 'NONE', ( #614 ), #14677, .F. ) ;
#9492=ORIENTED_EDGE ( 'NONE', *, *, #2600, .F. ) ;
#9493=ORIENTED_EDGE ( 'NONE', *, *, #21422, .T. ) ;
#9496=CARTESIAN_POINT ( 'NONE',  ( 50.62387473582167274, 34.52875999999999834, -28.41576006634952734 ) ) ;
#9499=VERTEX_POINT ( 'NONE', #12904 ) ;
#9500=CARTESIAN_POINT ( 'NONE',  ( 49.41195815393805901, 42.06303499999999929, -1.411525001868561224 ) ) ;
#9501=EDGE_CURVE ( 'NONE', #7839, #20066, #7900, .T. ) ;
#9508=AXIS2_PLACEMENT_3D ( 'NONE', #16199, #4791, #11523 ) ;
#9509=CARTESIAN_POINT ( 'NONE',  ( 52.69765441554997665, -7.547610000000001484, -16.33112036207927886 ) ) ;
#9516=CARTESIAN_POINT ( 'NONE',  ( 41.71184157647478230, 38.88803500000000213, -2.134205101306931862 ) ) ;
#9520=DIRECTION ( 'NONE',  ( 0.000000000000000000, 1.000000000000000000, 0.000000000000000000 ) ) ;
#9522=VECTOR ( 'NONE', #6929, 1000.000000000000000 ) ;
#9537=CARTESIAN_POINT ( 'NONE',  ( 38.46688692048027747, -5.391489964475852048, -4.537348303483145884 ) ) ;
#9544=EDGE_CURVE ( 'NONE', #5911, #14322, #9997, .T. ) ;
#9557=CARTESIAN_POINT ( 'NONE',  ( 47.80475250345343596, 38.88803500000000213, -11.91473563638196786 ) ) ;
#9558=ORIENTED_EDGE ( 'NONE', *, *, #16958, .T. ) ;
#9563=CIRCLE ( 'NONE', #18049, 30.16249999999999787 ) ;
#9569=ORIENTED_EDGE ( 'NONE', *, *, #14972, .T. ) ;
#9572=CLOSED_SHELL ( 'NONE', ( #8205, #9269, #5297, #10454, #21226, #11126, #21776, #9490, #12256, #2133, #2499, #6952, #6646, #8791, #3073, #18308, #2671, #16928, #718, #20848, #15915, #12254, #8388, #3242, #5966, #21406, #19078, #17019, #10900, #18023, #18304, #17352, #11549, #14098, #5201, #12381, #11955, #3685, #13179, #14072, #575, #12106, #6433, #182, #15843, #10632, #1245, #4926, #6229, #10051, #20093, #16932, #1383, #1613, #19384, #13879, #1536, #12889, #3374, #4563, #19646, #10032, #14820, #19769, #14839, #2418, #7981, #10576, #14113, #719, #850, #1166, #14347, #8577, #19797, #18330, #15023, #13039, #18536, #11960, #9385, #14798, #6295, #7658, #12654, #12902, #12467, #5880, #17238, #14049, #3817, #7136, #9887, #2043, #8500, #4423, #1193, #10873, #9673, #5426, #16355, #20113, #10879, #9645, #7509, #10383, #4139, #13093, #16560, #715, #13295, #7773, #7331, #11387, #18399, #18278, #8706, #19402, #8022, #21148, #15237, #17452, #3347, #12083, #8624, #20047, #11459, #2195, #6384, #1277, #6975, #17645, #4592, #13149, #2049, #20079, #11432, #9070, #15049, #21054, #13902, #9652, #20437, #9594, #4648, #13611, #16815, #4003 ) ) ;
#9574=EDGE_LOOP ( 'NONE', ( #21086, #6383, #7724, #15405 ) ) ;
#9575=AXIS2_PLACEMENT_3D ( 'NONE', #19007, #455, #661 ) ;
#9576=CARTESIAN_POINT ( 'NONE',  ( 34.72145145287101542, 2.586003464000000029, 0.5851394578805096947 ) ) ;
#9579=ORIENTED_EDGE ( 'NONE', *, *, #4364, .T. ) ;
#9582=CIRCLE ( 'NONE', #19460, 9.525000000000002132 ) ;
#9586=VECTOR ( 'NONE', #14815, 1000.000000000000000 ) ;
#9588=CIRCLE ( 'NONE', #21589, 0.5079999999999997851 ) ;
#9590=CARTESIAN_POINT ( 'NONE',  ( 39.93069333241970043, 38.72516837585681770, -3.008993689095889490 ) ) ;
#9594=ADVANCED_FACE ( 'NONE', ( #21278 ), #1265, .T. ) ;
#9595=AXIS2_PLACEMENT_3D ( 'NONE', #11593, #10250, #4948 ) ;
#9596=VECTOR ( 'NONE', #9757, 1000.000000000000000 ) ;
#9597=ORIENTED_EDGE ( 'NONE', *, *, #1777, .F. ) ;
#9603=ORIENTED_EDGE ( 'NONE', *, *, #10631, .F. ) ;
#9607=DIRECTION ( 'NONE',  ( 0.000000000000000000, 1.000000000000000000, 0.000000000000000000 ) ) ;
#9609=ORIENTED_EDGE ( 'NONE', *, *, #9501, .F. ) ;
#9610=VECTOR ( 'NONE', #7992, 1000.000000000000000 ) ;
#9611=ORIENTED_EDGE ( 'NONE', *, *, #454, .T. ) ;
#9612=DIRECTION ( 'NONE',  ( 0.5222415575336524229, 0.000000000000000000, 0.8527976052879281399 ) ) ;
#9614=VECTOR ( 'NONE', #392, 1000.000000000000114 ) ;
#9616=EDGE_CURVE ( 'NONE', #20092, #9393, #6134, .T. ) ;
#9617=CIRCLE ( 'NONE', #5052, 0.7950199999999985057 ) ;
#9624=CARTESIAN_POINT ( 'NONE',  ( 57.69402548289047417, 0.000000000000000000, -20.84562559047711261 ) ) ;
#9628=DIRECTION ( 'NONE',  ( 0.000000000000000000, -1.000000000000000000, -0.000000000000000000 ) ) ;
#9631=ORIENTED_EDGE ( 'NONE', *, *, #8761, .T. ) ;
#9637=DIRECTION ( 'NONE',  ( 0.000000000000000000, 1.000000000000000000, -0.000000000000000000 ) ) ;
#9645=ADVANCED_FACE ( 'NONE', ( #9769 ), #4588, .T. ) ;
#9646=CIRCLE ( 'NONE', #116, 30.16249999999999076 ) ;
#9652=ADVANCED_FACE ( 'NONE', ( #18080 ), #2940, .T. ) ;
#9653=CARTESIAN_POINT ( 'NONE',  ( 32.18388890846549799, 29.95901653600000003, 1.507793899792891468 ) ) ;
#9662=EDGE_LOOP ( 'NONE', ( #7208, #17310, #10739, #27 ) ) ;
#9665=DIRECTION ( 'NONE',  ( 0.000000000000000000, -1.000000000000000000, 0.000000000000000000 ) ) ;
#9667=CARTESIAN_POINT ( 'NONE',  ( 38.95211873669086344, -5.166601264346659228, -3.952980512833436322 ) ) ;
#9673=ADVANCED_FACE ( 'NONE', ( #21605 ), #6467, .T. ) ;
#9674=EDGE_CURVE ( 'NONE', #1021, #7959, #10989, .T. ) ;
#9680=AXIS2_PLACEMENT_3D ( 'NONE', #14760, #19917, #8088 ) ;
#9682=SURFACE_STYLE_USAGE ( .BOTH. , #11785 ) ;
#9686=AXIS2_PLACEMENT_3D ( 'NONE', #20481, #18838, #10447 ) ;
#9694=ORIENTED_EDGE ( 'NONE', *, *, #26, .F. ) ;
#9696=VECTOR ( 'NONE', #13921, 1000.000000000000000 ) ;
#9699=ORIENTED_EDGE ( 'NONE', *, *, #13846, .F. ) ;
#9703=DIRECTION ( 'NONE',  ( -0.4987171968201974948, 0.000000000000000000, 0.8667647648559581031 ) ) ;
#9706=ORIENTED_EDGE ( 'NONE', *, *, #9116, .F. ) ;
#9716=DIRECTION ( 'NONE',  ( 0.7421532822901579785, 0.000000000000000000, -0.6702301885068630005 ) ) ;
#9720=VERTEX_POINT ( 'NONE', #5224 ) ;
#9724=EDGE_CURVE ( 'NONE', #13886, #15003, #13653, .T. ) ;
#9728=DIRECTION ( 'NONE',  ( 0.000000000000000000, 1.000000000000000000, 0.000000000000000000 ) ) ;
#9732=ORIENTED_EDGE ( 'NONE', *, *, #15694, .F. ) ;
#9741=ORIENTED_EDGE ( 'NONE', *, *, #21259, .F. ) ;
#9743=CARTESIAN_POINT ( 'NONE',  ( 30.24348838687780727, 32.54502000000000095, -20.27293523655082552 ) ) ;
#9749=FACE_OUTER_BOUND ( 'NONE', #305, .T. ) ;
#9757=DIRECTION ( 'NONE',  ( 0.000000000000000000, 1.000000000000000000, 0.000000000000000000 ) ) ;
#9759=ORIENTED_EDGE ( 'NONE', *, *, #14971, .T. ) ;
#9760=DIRECTION ( 'NONE',  ( -0.2227372614607789347, 0.000000000000000000, -0.9748785115884710528 ) ) ;
#9761=EDGE_CURVE ( 'NONE', #97, #19859, #746, .T. ) ;
#9766=VECTOR ( 'NONE', #14995, 1000.000000000000114 ) ;
#9769=FACE_OUTER_BOUND ( 'NONE', #4959, .T. ) ;
#9770=EDGE_LOOP ( 'NONE', ( #19568, #2966, #3285, #3823 ) ) ;
#9771=CARTESIAN_POINT ( 'NONE',  ( 38.94885947252404179, -5.166721542084396823, -3.956611957468594287 ) ) ;
#9775=EDGE_CURVE ( 'NONE', #16183, #11029, #1400, .T. ) ;
#9777=ORIENTED_EDGE ( 'NONE', *, *, #2953, .F. ) ;
#9780=CARTESIAN_POINT ( 'NONE',  ( 38.86292893166786655, 40.07865999999999929, -4.051696374780784815 ) ) ;
#9787=DIRECTION ( 'NONE',  ( 0.000000000000000000, 1.000000000000000000, 0.000000000000000000 ) ) ;
#9788=ORIENTED_EDGE ( 'NONE', *, *, #7590, .T. ) ;
#9789=EDGE_CURVE ( 'NONE', #16977, #535, #146, .T. ) ;
#9791=EDGE_CURVE ( 'NONE', #15606, #9720, #20101, .T. ) ;
#9805=DIRECTION ( 'NONE',  ( -0.8667647648559581031, 0.000000000000000000, -0.4987171968201974948 ) ) ;
#9806=DIRECTION ( 'NONE',  ( 0.9129422336036122632, 0.000000000000000000, -0.4080888115384288528 ) ) ;
#9810=DIRECTION ( 'NONE',  ( 0.000000000000000000, -1.000000000000000000, -0.000000000000000000 ) ) ;
#9811=DIRECTION ( 'NONE',  ( 0.7532174416907898573, 0.000000000000000000, 0.6577716059034334206 ) ) ;
#9816=EDGE_CURVE ( 'NONE', #877, #9895, #11613, .T. ) ;
#9820=ORIENTED_EDGE ( 'NONE', *, *, #11578, .T. ) ;
#9822=CARTESIAN_POINT ( 'NONE',  ( 38.78586790977450960, 38.88803500000000213, -5.374168024304902147 ) ) ;
#9829=LINE ( 'NONE', #16599, #10150 ) ;
#9835=CARTESIAN_POINT ( 'NONE',  ( 42.35466991749225940, -9.531985000000000596, -17.94967221382040279 ) ) ;
#9837=EDGE_CURVE ( 'NONE', #5914, #4928, #9829, .T. ) ;
#9839=TOROIDAL_SURFACE ( 'NONE', #1716, 3.174999999999999822, 1.190625000000000044 ) ;
#9843=CARTESIAN_POINT ( 'NONE',  ( 46.03750000000000142, -9.531985000000000596, -10.31874999999999964 ) ) ;
#9864=ORIENTED_EDGE ( 'NONE', *, *, #570, .F. ) ;
#9866=AXIS2_PLACEMENT_3D ( 'NONE', #3939, #5910, #5580 ) ;
#9877=( GEOMETRIC_REPRESENTATION_CONTEXT ( 3 ) GLOBAL_UNCERTAINTY_ASSIGNED_CONTEXT ( ( #8771 ) ) GLOBAL_UNIT_ASSIGNED_CONTEXT ( ( #19730, #1382, #3280 ) ) REPRESENTATION_CONTEXT ( 'NONE', 'WORKASPACE' ) );
#9887=ADVANCED_FACE ( 'NONE', ( #19678 ), #4546, .F. ) ;
#9895=VERTEX_POINT ( 'NONE', #9624 ) ;
#9897=CARTESIAN_POINT ( 'NONE',  ( 61.65536943582333151, 0.000000000000000000, -11.98363747855214712 ) ) ;
#9905=VERTEX_POINT ( 'NONE', #8185 ) ;
#9908=PLANE ( 'NONE',  #19888 ) ;
#9925=CARTESIAN_POINT ( 'NONE',  ( 36.73521423675246922, 0.000000000000000000, 2.413462327205186497 ) ) ;
#9929=AXIS2_PLACEMENT_3D ( 'NONE', #1306, #11156, #19655 ) ;
#9931=DIRECTION ( 'NONE',  ( 0.000000000000000000, 0.000000000000000000, -1.000000000000000000 ) ) ;
#9934=AXIS2_PLACEMENT_3D ( 'NONE', #12869, #16889, #4456 ) ;
#9937=ORIENTED_EDGE ( 'NONE', *, *, #2744, .F. ) ;
#9943=EDGE_CURVE ( 'NONE', #14493, #1074, #6623, .T. ) ;
#9945=PLANE ( 'NONE',  #16594 ) ;
#9950=CARTESIAN_POINT ( 'NONE',  ( 59.55063415577301811, 0.000000000000000000, -22.52230776719629191 ) ) ;
#9951=VERTEX_POINT ( 'NONE', #3536 ) ;
#9964=VECTOR ( 'NONE', #1527, 1000.000000000000114 ) ;
#9968=DIRECTION ( 'NONE',  ( -0.6702301885068632226, 0.000000000000000000, -0.7421532822901576454 ) ) ;
#9970=CARTESIAN_POINT ( 'NONE',  ( 30.25543876212147509, -1.983739999999999837, -19.39939755251907272 ) ) ;
#9973=EDGE_CURVE ( 'NONE', #16183, #2705, #8499, .T. ) ;
#9976=CARTESIAN_POINT ( 'NONE',  ( 38.18512253410862201, -6.356984999999999886, -4.927479914652648674 ) ) ;
#9978=CYLINDRICAL_SURFACE ( 'NONE', #13913, 1.190624999999997824 ) ;
#9979=VECTOR ( 'NONE', #1038, 1000.000000000000000 ) ;
#9980=AXIS2_PLACEMENT_3D ( 'NONE', #17772, #10575, #11016 ) ;
#9981=DIRECTION ( 'NONE',  ( 0.1060008583745199739, 0.000000000000000000, 0.9943660382494290406 ) ) ;
#9983=CARTESIAN_POINT ( 'NONE',  ( 46.07940063401251507, -1.983739999999999837, -26.08707253294707229 ) ) ;
#9987=DIRECTION ( 'NONE',  ( 0.000000000000000000, 1.000000000000000000, 0.000000000000000000 ) ) ;
#9988=B_SPLINE_CURVE_WITH_KNOTS ( 'NONE', 3,
 ( #12899, #14443, #14341, #5907, #1042 ),
 .UNSPECIFIED., .F., .F.,
 ( 4, 1, 4 ),
 ( 0.007480389903054724364, 0.007494994329911808424, 0.007509598756768892484 ),
 .UNSPECIFIED. ) ;
#9997=LINE ( 'NONE', #11447, #2163 ) ;
#9998=ORIENTED_EDGE ( 'NONE', *, *, #20311, .T. ) ;
#10007=AXIS2_PLACEMENT_3D ( 'NONE', #11311, #6444, #17953 ) ;
#10009=FACE_OUTER_BOUND ( 'NONE', #2662, .T. ) ;
#10012=FILL_AREA_STYLE_COLOUR ( '', #18360 ) ;
#10014=ORIENTED_EDGE ( 'NONE', *, *, #2395, .T. ) ;
#10020=CARTESIAN_POINT ( 'NONE',  ( 37.51913901087312553, -9.531985000000000596, -14.58057485080488114 ) ) ;
#10022=DIRECTION ( 'NONE',  ( 0.000000000000000000, -1.000000000000000000, -0.000000000000000000 ) ) ;
#10023=ORIENTED_EDGE ( 'NONE', *, *, #13846, .T. ) ;
#10030=DIRECTION ( 'NONE',  ( -0.8943161143440100380, 0.000000000000000000, -0.4474356798743612806 ) ) ;
#10031=EDGE_LOOP ( 'NONE', ( #6564, #3756, #13128, #1571 ) ) ;
#10032=ADVANCED_FACE ( 'NONE', ( #5185 ), #12052, .F. ) ;
#10036=DIRECTION ( 'NONE',  ( -0.000000000000000000, -1.000000000000000000, 0.000000000000000000 ) ) ;
#10038=CARTESIAN_POINT ( 'NONE',  ( 39.37934099661365650, 40.07865999999999929, -4.303499184870370975 ) ) ;
#10040=ORIENTED_EDGE ( 'NONE', *, *, #11997, .F. ) ;
#10041=DIRECTION ( 'NONE',  ( 0.6702301885068628895, 0.000000000000000000, 0.7421532822901579785 ) ) ;
#10042=DIRECTION ( 'NONE',  ( 0.000000000000000000, 1.000000000000000000, 0.000000000000000000 ) ) ;
#10045=ORIENTED_EDGE ( 'NONE', *, *, #7163, .F. ) ;
#10051=ADVANCED_FACE ( 'NONE', ( #106 ), #10499, .F. ) ;
#10054=ORIENTED_EDGE ( 'NONE', *, *, #14354, .T. ) ;
#10060=CYLINDRICAL_SURFACE ( 'NONE', #521, 30.16250000000000142 ) ;
#10065=CARTESIAN_POINT ( 'NONE',  ( 44.27024749654614055, -6.356984999999999886, -8.722764363618502159 ) ) ;
#10066=DIRECTION ( 'NONE',  ( -0.2227372614607789347, 0.000000000000000000, -0.9748785115884710528 ) ) ;
#10075=EDGE_CURVE ( 'NONE', #14810, #7476, #11936, .T. ) ;
#10077=PLANE ( 'NONE',  #2809 ) ;
#10078=CARTESIAN_POINT ( 'NONE',  ( 34.38097451710952868, -1.983739999999999837, 0.2081255904771098786 ) ) ;
#10082=CIRCLE ( 'NONE', #5136, 30.16250000000000497 ) ;
#10089=DIRECTION ( 'NONE',  ( -0.9129422336036122632, 0.000000000000000000, 0.4080888115384288528 ) ) ;
#10090=CARTESIAN_POINT ( 'NONE',  ( 39.00487391863466513, 40.07742955315917044, -3.894748490060887747 ) ) ;
#10092=CYLINDRICAL_SURFACE ( 'NONE', #16288, 0.5080000000000006732 ) ;
#10096=VERTEX_POINT ( 'NONE', #5286 ) ;
#10117=CIRCLE ( 'NONE', #4480, 1.190624999999997824 ) ;
#10129=ORIENTED_EDGE ( 'NONE', *, *, #20187, .F. ) ;
#10131=ORIENTED_EDGE ( 'NONE', *, *, #2872, .T. ) ;
#10134=VERTEX_POINT ( 'NONE', #2313 ) ;
#10135=FACE_OUTER_BOUND ( 'NONE', #3085, .T. ) ;
#10136=DIRECTION ( 'NONE',  ( 0.000000000000000000, 1.000000000000000000, 0.000000000000000000 ) ) ;
#10137=LINE ( 'NONE', #8586, #3372 ) ;
#10142=DIRECTION ( 'NONE',  ( 0.000000000000000000, 1.000000000000000000, 0.000000000000000000 ) ) ;
#10143=DIRECTION ( 'NONE',  ( 0.3542738219355897056, 0.000000000000000000, 0.9351417320872542627 ) ) ;
#10146=VERTEX_POINT ( 'NONE', #6361 ) ;
#10147=EDGE_LOOP ( 'NONE', ( #8710, #5760, #13724, #9144, #6572, #16477, #7524, #21350, #2880, #3250, #20102, #8061, #9611, #5279, #8804, #21456, #7951, #17568, #12644, #14913, #21389, #5498, #14826, #3060, #14045, #20376, #11389, #12503, #5392, #6839, #16154, #312, #9415, #838, #1283, #13343, #2544, #5837, #16247, #18081 ) ) ;
#10150=VECTOR ( 'NONE', #18034, 1000.000000000000000 ) ;
#10152=VERTEX_POINT ( 'NONE', #14692 ) ;
#10160=CYLINDRICAL_SURFACE ( 'NONE', #7214, 1.190624999999999822 ) ;
#10169=CARTESIAN_POINT ( 'NONE',  ( 52.59626903419218280, -5.404081211114977634, -17.22676038219739780 ) ) ;
#10170=DIRECTION ( 'NONE',  ( 0.000000000000000000, 1.000000000000000000, 0.000000000000000000 ) ) ;
#10180=DIRECTION ( 'NONE',  ( 0.000000000000000000, 1.000000000000000000, 0.000000000000000000 ) ) ;
#10190=CARTESIAN_POINT ( 'NONE',  ( 36.80301088673436283, 34.52875999999999834, -23.10021947667301134 ) ) ;
#10194=CARTESIAN_POINT ( 'NONE',  ( 49.72033008250774344, 42.06303499999999929, -2.687827786179598277 ) ) ;
#10196=CARTESIAN_POINT ( 'NONE',  ( 37.09580597189848561, 38.88803500000000213, 2.672127428255844261 ) ) ;
#10200=DIRECTION ( 'NONE',  ( -0.9987059298363657467, 0.000000000000000000, -0.05085730733808409287 ) ) ;
#10209=FACE_OUTER_BOUND ( 'NONE', #3477, .T. ) ;
#10225=ORIENTED_EDGE ( 'NONE', *, *, #20018, .F. ) ;
#10237=CARTESIAN_POINT ( 'NONE',  ( 32.42378190387104553, 32.54502000000000095, -18.15178106273469183 ) ) ;
#10238=ORIENTED_EDGE ( 'NONE', *, *, #18355, .T. ) ;
#10243=CYLINDRICAL_SURFACE ( 'NONE', #15658, 0.5079999999999996740 ) ;
#10249=DIRECTION ( 'NONE',  ( 0.000000000000000000, -1.000000000000000000, -0.000000000000000000 ) ) ;
#10250=DIRECTION ( 'NONE',  ( 0.000000000000000000, 1.000000000000000000, 0.000000000000000000 ) ) ;
#10255=ORIENTED_EDGE ( 'NONE', *, *, #18942, .F. ) ;
#10261=ORIENTED_EDGE ( 'NONE', *, *, #5242, .T. ) ;
#10263=ORIENTED_EDGE ( 'NONE', *, *, #2738, .F. ) ;
#10264=VECTOR ( 'NONE', #2597, 1000.000000000000000 ) ;
#10270=AXIS2_PLACEMENT_3D ( 'NONE', #6784, #8755, #13432 ) ;
#10271=DIRECTION ( 'NONE',  ( 0.9987059298363657467, 0.000000000000000000, 0.05085730733808445370 ) ) ;
#10276=DIRECTION ( 'NONE',  ( -0.7421532822901562021, 0.000000000000000000, 0.6702301885068651099 ) ) ;
#10277=DIRECTION ( 'NONE',  ( -0.9784543669157950152, 0.000000000000000000, -0.2064631973582961577 ) ) ;
#10278=CARTESIAN_POINT ( 'NONE',  ( 45.99559936598748777, -1.983739999999999837, 5.449572532947073000 ) ) ;
#10279=CARTESIAN_POINT ( 'NONE',  ( 41.78116128337411794, 0.000000000000000000, 7.392073290253172502 ) ) ;
#10286=ORIENTED_EDGE ( 'NONE', *, *, #21101, .F. ) ;
#10292=EDGE_CURVE ( 'NONE', #8259, #4430, #10705, .T. ) ;
#10297=DIRECTION ( 'NONE',  ( -0.9784543669157947932, 0.000000000000000000, -0.2064631973582977953 ) ) ;
#10304=DIRECTION ( 'NONE',  ( 0.7421532822901579785, -0.000000000000000000, -0.6702301885068630005 ) ) ;
#10307=DIRECTION ( 'NONE',  ( 0.000000000000000000, 1.000000000000000000, 0.000000000000000000 ) ) ;
#10313=VECTOR ( 'NONE', #17143, 1000.000000000000000 ) ;
#10326=AXIS2_PLACEMENT_3D ( 'NONE', #3251, #11975, #15197 ) ;
#10328=ORIENTED_EDGE ( 'NONE', *, *, #16837, .F. ) ;
#10329=CIRCLE ( 'NONE', #18437, 9.525000000000002132 ) ;
#10338=EDGE_CURVE ( 'NONE', #14783, #1582, #268, .T. ) ;
#10340=CARTESIAN_POINT ( 'NONE',  ( 39.11079947626275555, -1.983739999999999837, -27.65534212225540500 ) ) ;
#10348=CARTESIAN_POINT ( 'NONE',  ( 55.33978576324753362, 32.54502000000000095, -23.05096232720518756 ) ) ;
#10352=EDGE_CURVE ( 'NONE', #16343, #8304, #21295, .T. ) ;
#10357=CIRCLE ( 'NONE', #18129, 0.5080000000000012284 ) ;
#10363=DIRECTION ( 'NONE',  ( 0.000000000000000000, 1.000000000000000000, -0.000000000000000000 ) ) ;
#10366=CARTESIAN_POINT ( 'NONE',  ( 59.55063415577301811, -1.983739999999999837, -22.52230776719629191 ) ) ;
#10368=DIRECTION ( 'NONE',  ( 0.000000000000000000, 0.000000000000000000, -1.000000000000000000 ) ) ;
#10371=CARTESIAN_POINT ( 'NONE',  ( 46.03750000000000142, 32.54502000000000095, -10.31874999999999964 ) ) ;
#10381=B_SPLINE_CURVE_WITH_KNOTS ( 'NONE', 3,
 ( #7353, #15889, #12332, #12666 ),
 .UNSPECIFIED., .F., .F.,
 ( 4, 4 ),
 ( -7.968845587669719102E-05, 0.0005316928842662705084 ),
 .UNSPECIFIED. ) ;
#10383=ADVANCED_FACE ( 'NONE', ( #1887 ), #3667, .F. ) ;
#10384=DIRECTION ( 'NONE',  ( 0.8943161143440100380, 0.000000000000000000, 0.4474356798743612806 ) ) ;
#10394=CARTESIAN_POINT ( 'NONE',  ( 27.40895291499714403, 34.52875999999999834, -9.088367920799473865 ) ) ;
#10399=DIRECTION ( 'NONE',  ( -0.7421532822901579785, -0.000000000000000000, 0.6702301885068630005 ) ) ;
#10400=CARTESIAN_POINT ( 'NONE',  ( 48.78323016782857735, 0.000000000000000000, -25.79158832643865651 ) ) ;
#10403=CARTESIAN_POINT ( 'NONE',  ( 43.29176983217143260, -1.983739999999999837, 5.154088326438659884 ) ) ;
#10405=EDGE_LOOP ( 'NONE', ( #7083, #17250, #16868, #404 ) ) ;
#10406=VECTOR ( 'NONE', #5402, 1000.000000000000000 ) ;
#10407=CYLINDRICAL_SURFACE ( 'NONE', #3891, 9.524999999999998579 ) ;
#10409=EDGE_CURVE ( 'NONE', #11247, #10898, #16725, .T. ) ;
#10416=FACE_OUTER_BOUND ( 'NONE', #19945, .T. ) ;
#10419=CIRCLE ( 'NONE', #14709, 30.16249999999999076 ) ;
#10424=LINE ( 'NONE', #13321, #11309 ) ;
#10425=DIRECTION ( 'NONE',  ( 0.07875956036501312318, 0.000000000000000000, -0.9968936410927243807 ) ) ;
#10426=CARTESIAN_POINT ( 'NONE',  ( 50.29383871662588490, 29.95901653600000003, -28.02957329025317179 ) ) ;
#10432=EDGE_CURVE ( 'NONE', #3770, #7380, #10530, .T. ) ;
#10433=LINE ( 'NONE', #15534, #673 ) ;
#10442=ORIENTED_EDGE ( 'NONE', *, *, #2744, .T. ) ;
#10447=DIRECTION ( 'NONE',  ( 0.9959941601142464629, 0.000000000000000000, 0.08941830359784717908 ) ) ;
#10451=EDGE_LOOP ( 'NONE', ( #2321, #21768, #14071 ) ) ;
#10454=ADVANCED_FACE ( 'NONE', ( #3346 ), #3463, .T. ) ;
#10461=ORIENTED_EDGE ( 'NONE', *, *, #18858, .F. ) ;
#10463=VERTEX_POINT ( 'NONE', #10078 ) ;
#10466=DIRECTION ( 'NONE',  ( -0.8943161143440100380, 0.000000000000000000, -0.4474356798743612806 ) ) ;
#10469=DIRECTION ( 'NONE',  ( -0.7532174416907910786, 0.000000000000000000, -0.6577716059034319773 ) ) ;
#10470=PLANE ( 'NONE',  #9437 ) ;
#10472=ORIENTED_EDGE ( 'NONE', *, *, #11011, .T. ) ;
#10475=CARTESIAN_POINT ( 'NONE',  ( 52.44708915697334106, 0.000000000000000000, 4.020247972991190188 ) ) ;
#10480=VERTEX_POINT ( 'NONE', #12071 ) ;
#10483=DIRECTION ( 'NONE',  ( 0.000000000000000000, -1.000000000000000000, -0.000000000000000000 ) ) ;
#10488=VECTOR ( 'NONE', #5012, 1000.000000000000000 ) ;
#10496=LINE ( 'NONE', #16905, #10406 ) ;
#10499=CYLINDRICAL_SURFACE ( 'NONE', #1323, 0.5079999999999996740 ) ;
#10504=CARTESIAN_POINT ( 'NONE',  ( 52.25302947726946456, -6.201940431049069780, -17.53628547414362515 ) ) ;
#10505=CARTESIAN_POINT ( 'NONE',  ( 32.10373694497760511, -6.356984999999999886, -3.785462747693984831 ) ) ;
#10506=EDGE_LOOP ( 'NONE', ( #21853, #19178, #16864, #9788 ) ) ;
#10508=CARTESIAN_POINT ( 'NONE',  ( 54.61912012054379062, -6.356984999999999886, -13.79062155615056362 ) ) ;
#10517=CARTESIAN_POINT ( 'NONE',  ( 38.98667580346275940, 40.07845397843726687, -3.914708526915718689 ) ) ;
#10519=LINE ( 'NONE', #2339, #9310 ) ;
#10527=DIRECTION ( 'NONE',  ( 0.9237641507921645623, 0.000000000000000000, 0.3829618697876213673 ) ) ;
#10529=DIRECTION ( 'NONE',  ( -0.7421532822901572013, 0.000000000000000000, 0.6702301885068637777 ) ) ;
#10530=CIRCLE ( 'NONE', #11931, 0.5080000000000001181 ) ;
#10531=FACE_OUTER_BOUND ( 'NONE', #9770, .T. ) ;
#10541=CARTESIAN_POINT ( 'NONE',  ( 64.66604708500285881, 32.54502000000000095, -11.54913207920052720 ) ) ;
#10543=VERTEX_POINT ( 'NONE', #568 ) ;
#10554=ORIENTED_EDGE ( 'NONE', *, *, #1060, .T. ) ;
#10564=VERTEX_POINT ( 'NONE', #19015 ) ;
#10568=VERTEX_POINT ( 'NONE', #7212 ) ;
#10575=DIRECTION ( 'NONE',  ( -0.7421532822901579785, 0.000000000000000000, 0.6702301885068630005 ) ) ;
#10576=ADVANCED_FACE ( 'NONE', ( #3890 ), #2446, .T. ) ;
#10579=DIRECTION ( 'NONE',  ( -0.000000000000000000, -1.000000000000000000, 0.000000000000000000 ) ) ;
#10580=CARTESIAN_POINT ( 'NONE',  ( 32.16428892652708527, -6.356984999999999886, -4.974546995406843308 ) ) ;
#10583=AXIS2_PLACEMENT_3D ( 'NONE', #2052, #10136, #11908 ) ;
#10584=DIRECTION ( 'NONE',  ( 0.7421532822901579785, 0.000000000000000000, -0.6702301885068628895 ) ) ;
#10587=LINE ( 'NONE', #5166, #4209 ) ;
#10589=ORIENTED_EDGE ( 'NONE', *, *, #19696, .T. ) ;
#10590=ORIENTED_EDGE ( 'NONE', *, *, #16837, .T. ) ;
#10597=EDGE_LOOP ( 'NONE', ( #18246, #13716, #19560, #17375, #5009, #19640 ) ) ;
#10598=VECTOR ( 'NONE', #14447, 1000.000000000000114 ) ;
#10599=ORIENTED_EDGE ( 'NONE', *, *, #11055, .F. ) ;
#10602=ORIENTED_EDGE ( 'NONE', *, *, #2511, .T. ) ;
#10604=VECTOR ( 'NONE', #15444, 1000.000000000000000 ) ;
#10606=EDGE_CURVE ( 'NONE', #21599, #7998, #9288, .T. ) ;
#10608=CARTESIAN_POINT ( 'NONE',  ( 38.32938179974708959, -7.102284129468043439, -4.721977392770211779 ) ) ;
#10611=CARTESIAN_POINT ( 'NONE',  ( 61.60152099976809126, 37.11476346399999926, -12.48877542598203405 ) ) ;
#10612=CIRCLE ( 'NONE', #1075, 1.190625000000000711 ) ;
#10614=CARTESIAN_POINT ( 'NONE',  ( 48.78323016782857735, -1.983739999999999837, -25.79158832643865651 ) ) ;
#10616=DIRECTION ( 'NONE',  ( 0.000000000000000000, -1.000000000000000000, 0.000000000000000000 ) ) ;
#10618=ORIENTED_EDGE ( 'NONE', *, *, #12304, .F. ) ;
#10631=EDGE_CURVE ( 'NONE', #9499, #18470, #2332, .T. ) ;
#10632=ADVANCED_FACE ( 'NONE', ( #12185 ), #9171, .F. ) ;
#10637=AXIS2_PLACEMENT_3D ( 'NONE', #2462, #14415, #17723 ) ;
#10660=EDGE_CURVE ( 'NONE', #9895, #11597, #14078, .T. ) ;
#10661=LINE ( 'NONE', #373, #867 ) ;
#10663=TOROIDAL_SURFACE ( 'NONE', #1808, 3.174999999999999822, 1.190625000000000044 ) ;
#10670=CIRCLE ( 'NONE', #3252, 30.16250000000000497 ) ;
#10671=DIRECTION ( 'NONE',  ( 0.000000000000000000, -1.000000000000000000, 0.000000000000000000 ) ) ;
#10688=FACE_OUTER_BOUND ( 'NONE', #4156, .T. ) ;
#10690=CIRCLE ( 'NONE', #8213, 9.524999999999996803 ) ;
#10694=DIRECTION ( 'NONE',  ( 0.000000000000000000, -1.000000000000000000, -0.000000000000000000 ) ) ;
#10698=LINE ( 'NONE', #18970, #5186 ) ;
#10701=CARTESIAN_POINT ( 'NONE',  ( 60.38511073144201191, -1.983739999999999837, -22.26373525985038526 ) ) ;
#10704=FACE_BOUND ( 'NONE', #2470, .T. ) ;
#10705=LINE ( 'NONE', #12810, #2396 ) ;
#10709=LINE ( 'NONE', #15482, #12439 ) ;
#10716=VERTEX_POINT ( 'NONE', #2101 ) ;
#10717=EDGE_CURVE ( 'NONE', #14160, #5388, #21220, .T. ) ;
#10721=DIRECTION ( 'NONE',  ( 0.000000000000000000, 1.000000000000000000, 0.000000000000000000 ) ) ;
#10724=CARTESIAN_POINT ( 'NONE',  ( 54.72004008979249789, -6.356984999999999886, -15.77242863567076014 ) ) ;
#10732=FACE_OUTER_BOUND ( 'NONE', #6304, .T. ) ;
#10734=ORIENTED_EDGE ( 'NONE', *, *, #498, .T. ) ;
#10739=ORIENTED_EDGE ( 'NONE', *, *, #17168, .F. ) ;
#10742=CARTESIAN_POINT ( 'NONE',  ( 54.61912012054379062, -6.356984999999999886, -13.79062155615056362 ) ) ;
#10755=DIRECTION ( 'NONE',  ( 0.000000000000000000, 0.000000000000000000, 1.000000000000000000 ) ) ;
#10758=EDGE_CURVE ( 'NONE', #9392, #13313, #14503, .T. ) ;
#10759=CIRCLE ( 'NONE', #21687, 9.525000000000002132 ) ;
#10761=DIRECTION ( 'NONE',  ( 0.7421532822901579785, 0.000000000000000000, -0.6702301885068630005 ) ) ;
#10762=EDGE_CURVE ( 'NONE', #15942, #3338, #13794, .T. ) ;
#10766=DIRECTION ( 'NONE',  ( 0.000000000000000000, -1.000000000000000000, -0.000000000000000000 ) ) ;
#10772=VERTEX_POINT ( 'NONE', #11903 ) ;
#10778=CARTESIAN_POINT ( 'NONE',  ( 46.03750000000000142, 42.06303499999999929, -10.31874999999999964 ) ) ;
#10783=DIRECTION ( 'NONE',  ( -0.3928209820863007296, 0.000000000000000000, 0.9196149607486571176 ) ) ;
#10791=DIRECTION ( 'NONE',  ( 0.000000000000000000, 1.000000000000000000, -0.000000000000000000 ) ) ;
#10794=ORIENTED_EDGE ( 'NONE', *, *, #20187, .T. ) ;
#10797=CARTESIAN_POINT ( 'NONE',  ( 39.70735255319233659, -6.957959099329872998, -3.201272008584183482 ) ) ;
#10801=EDGE_LOOP ( 'NONE', ( #2391, #20208, #18629, #15703 ) ) ;
#10802=LINE ( 'NONE', #21068, #8554 ) ;
#10812=VERTEX_POINT ( 'NONE', #12342 ) ;
#10833=VERTEX_POINT ( 'NONE', #20384 ) ;
#10836=CIRCLE ( 'NONE', #3784, 1.190625000000000711 ) ;
#10838=CARTESIAN_POINT ( 'NONE',  ( 32.10373694497760511, -6.356984999999999886, -3.785462747693984831 ) ) ;
#10847=CYLINDRICAL_SURFACE ( 'NONE', #5775, 0.5079999999999963434 ) ;
#10849=AXIS2_PLACEMENT_3D ( 'NONE', #14144, #17659, #12806 ) ;
#10858=DIRECTION ( 'NONE',  ( 0.9959941601142464629, 0.000000000000000000, 0.08941830359784661009 ) ) ;
#10861=ORIENTED_EDGE ( 'NONE', *, *, #19953, .F. ) ;
#10872=CARTESIAN_POINT ( 'NONE',  ( 38.94885947252247860, -7.547248457916676756, -3.956611957470116625 ) ) ;
#10873=ADVANCED_FACE ( 'NONE', ( #2161 ), #8905, .F. ) ;
#10878=DIRECTION ( 'NONE',  ( -0.7421532822901572013, 0.000000000000000000, 0.6702301885068637777 ) ) ;
#10879=ADVANCED_FACE ( 'NONE', ( #10688 ), #619, .T. ) ;
#10880=DIRECTION ( 'NONE',  ( -0.9784543669157944601, 0.000000000000000000, -0.2064631973582987667 ) ) ;
#10882=CARTESIAN_POINT ( 'NONE',  ( 59.80894853325292360, -6.356984999999999886, -16.70545285374888778 ) ) ;
#10887=CARTESIAN_POINT ( 'NONE',  ( 52.29466199406144966, 39.42598491866655763, -17.50029076404656792 ) ) ;
#10894=ORIENTED_EDGE ( 'NONE', *, *, #20692, .T. ) ;
#10898=VERTEX_POINT ( 'NONE', #5705 ) ;
#10900=ADVANCED_FACE ( 'NONE', ( #2717 ), #19296, .T. ) ;
#10921=ORIENTED_EDGE ( 'NONE', *, *, #8673, .T. ) ;
#10925=EDGE_CURVE ( 'NONE', #3091, #20317, #16571, .T. ) ;
#10926=AXIS2_PLACEMENT_3D ( 'NONE', #20718, #2267, #5572 ) ;
#10931=DIRECTION ( 'NONE',  ( 0.9959941601142464629, 0.000000000000000000, 0.08941830359784717908 ) ) ;
#10941=DIRECTION ( 'NONE',  ( 0.1060008583745200711, 0.000000000000000000, 0.9943660382494290406 ) ) ;
#10944=EDGE_LOOP ( 'NONE', ( #9379, #20073, #17255, #2046 ) ) ;
#10945=CARTESIAN_POINT ( 'NONE',  ( 61.09555596642878328, 0.000000000000000000, -12.53419992421059348 ) ) ;
#10957=AXIS2_PLACEMENT_3D ( 'NONE', #20892, #4534, #12518 ) ;
#10972=EDGE_LOOP ( 'NONE', ( #15723, #866, #21740, #20527, #10602, #19216 ) ) ;
#10982=DIRECTION ( 'NONE',  ( 0.7421532822901579785, 0.000000000000000000, -0.6702301885068628895 ) ) ;
#10987=CARTESIAN_POINT ( 'NONE',  ( 41.78116128337411794, -1.983739999999999837, 7.392073290253172502 ) ) ;
#10989=CIRCLE ( 'NONE', #2110, 0.5080000000000013394 ) ;
#10990=CARTESIAN_POINT ( 'NONE',  ( 41.45112526417833010, 32.54502000000000095, 7.778260066349530710 ) ) ;
#10991=CARTESIAN_POINT ( 'NONE',  ( 64.19677489640052670, -4.569743463999999200, -11.74367670905533423 ) ) ;
#10994=CARTESIAN_POINT ( 'NONE',  ( 61.02111788801703085, -1.983739999999999837, -5.406220493519755088 ) ) ;
#10995=VERTEX_POINT ( 'NONE', #4385 ) ;
#10997=LINE ( 'NONE', #9107, #20428 ) ;
#11001=CARTESIAN_POINT ( 'NONE',  ( 42.94469661997857912, -76.79125307200000350, -18.48251861828712705 ) ) ;
#11006=VECTOR ( 'NONE', #21035, 1000.000000000000000 ) ;
#11007=CARTESIAN_POINT ( 'NONE',  ( 39.18191486213413555, -5.198066315796270764, -3.704589387597398087 ) ) ;
#11009=AXIS2_PLACEMENT_3D ( 'NONE', #1610, #11790, #3388 ) ;
#11011=EDGE_CURVE ( 'NONE', #14493, #14322, #3149, .T. ) ;
#11016=DIRECTION ( 'NONE',  ( 0.000000000000000000, -1.000000000000000000, 0.000000000000000000 ) ) ;
#11024=EDGE_CURVE ( 'NONE', #17175, #1068, #15006, .T. ) ;
#11025=CARTESIAN_POINT ( 'NONE',  ( 42.79471501377724252, 0.000000000000000000, 5.049205022181460834 ) ) ;
#11029=VERTEX_POINT ( 'NONE', #21723 ) ;
#11030=CIRCLE ( 'NONE', #3611, 1.190625000000001155 ) ;
#11033=DIRECTION ( 'NONE',  ( -0.8943161143440100380, 0.000000000000000000, -0.4474356798743607255 ) ) ;
#11036=ORIENTED_EDGE ( 'NONE', *, *, #3794, .F. ) ;
#11039=EDGE_LOOP ( 'NONE', ( #5946, #4178, #8362, #19372 ) ) ;
#11041=AXIS2_PLACEMENT_3D ( 'NONE', #14994, #21711, #4582 ) ;
#11049=CARTESIAN_POINT ( 'NONE',  ( 38.82016491058538321, -1.983739999999999837, -14.75770094105646812 ) ) ;
#11055=EDGE_CURVE ( 'NONE', #1512, #968, #2824, .T. ) ;
#11061=ORIENTED_EDGE ( 'NONE', *, *, #19696, .F. ) ;
#11063=DIRECTION ( 'NONE',  ( 0.000000000000000000, -1.000000000000000000, -0.000000000000000000 ) ) ;
#11085=CARTESIAN_POINT ( 'NONE',  ( 53.00421038040393995, 29.95901653600000003, 6.511420152579801446 ) ) ;
#11089=CIRCLE ( 'NONE', #1544, 0.7950199999999982836 ) ;
#11102=CARTESIAN_POINT ( 'NONE',  ( 39.07078961959606289, 29.95901653600000003, -27.14892015257980162 ) ) ;
#11110=DIRECTION ( 'NONE',  ( 0.000000000000000000, -1.000000000000000000, -0.000000000000000000 ) ) ;
#11118=CIRCLE ( 'NONE', #1574, 1.190624999999997824 ) ;
#11119=PLANE ( 'NONE',  #7452 ) ;
#11120=CARTESIAN_POINT ( 'NONE',  ( 39.38402901577369875, -5.317104264161899074, -3.501309714141658258 ) ) ;
#11124=ORIENTED_EDGE ( 'NONE', *, *, #20699, .T. ) ;
#11126=ADVANCED_FACE ( 'NONE', ( #10209 ), #13769, .T. ) ;
#11132=ORIENTED_EDGE ( 'NONE', *, *, #10338, .T. ) ;
#11133=EDGE_CURVE ( 'NONE', #1512, #7380, #16953, .T. ) ;
#11137=ORIENTED_EDGE ( 'NONE', *, *, #2372, .T. ) ;
#11144=VERTEX_POINT ( 'NONE', #17068 ) ;
#11146=CIRCLE ( 'NONE', #1603, 0.5080000000000000071 ) ;
#11152=LINE ( 'NONE', #12940, #7917 ) ;
#11154=EDGE_LOOP ( 'NONE', ( #4711, #412, #18509, #9579 ) ) ;
#11155=DIRECTION ( 'NONE',  ( 0.6702301885068638887, 0.000000000000000000, 0.7421532822901570903 ) ) ;
#11156=DIRECTION ( 'NONE',  ( 0.000000000000000000, -1.000000000000000000, -0.000000000000000000 ) ) ;
#11168=DIRECTION ( 'NONE',  ( -0.000000000000000000, -1.000000000000000000, 0.000000000000000000 ) ) ;
#11177=DIRECTION ( 'NONE',  ( 0.000000000000000000, -1.000000000000000000, -0.000000000000000000 ) ) ;
#11183=DIRECTION ( 'NONE',  ( 0.7532174416907910786, 0.000000000000000000, 0.6577716059034319773 ) ) ;
#11187=DIRECTION ( 'NONE',  ( -0.6702301885068628895, 0.000000000000000000, -0.7421532822901579785 ) ) ;
#11189=ORIENTED_EDGE ( 'NONE', *, *, #19135, .F. ) ;
#11193=CARTESIAN_POINT ( 'NONE',  ( 49.79678389823170903, -1.983739999999999837, -28.13445659451038594 ) ) ;
#11199=ORIENTED_EDGE ( 'NONE', *, *, #286, .F. ) ;
#11204=CARTESIAN_POINT ( 'NONE',  ( 38.27578610983103857, -5.744908453443699159, -4.797394063557049115 ) ) ;
#11206=DIRECTION ( 'NONE',  ( 0.000000000000000000, 1.000000000000000000, 0.000000000000000000 ) ) ;
#11207=DIRECTION ( 'NONE',  ( 0.000000000000000000, 1.000000000000000000, -0.000000000000000000 ) ) ;
#11211=VECTOR ( 'NONE', #17138, 1000.000000000000000 ) ;
#11213=DIRECTION ( 'NONE',  ( 0.000000000000000000, 1.000000000000000000, 0.000000000000000000 ) ) ;
#11214=FACE_OUTER_BOUND ( 'NONE', #7600, .T. ) ;
#11222=DIRECTION ( 'NONE',  ( 0.000000000000000000, 1.000000000000000000, 0.000000000000000000 ) ) ;
#11223=VERTEX_POINT ( 'NONE', #1914 ) ;
#11230=CARTESIAN_POINT ( 'NONE',  ( 37.51913901087312553, 34.52875999999999834, -14.58057485080488114 ) ) ;
#11242=CYLINDRICAL_SURFACE ( 'NONE', #12035, 1.190625000000000711 ) ;
#11243=ORIENTED_EDGE ( 'NONE', *, *, #15074, .F. ) ;
#11247=VERTEX_POINT ( 'NONE', #20005 ) ;
#11249=EDGE_CURVE ( 'NONE', #5690, #12990, #20780, .T. ) ;
#11252=AXIS2_PLACEMENT_3D ( 'NONE', #7026, #15684, #512 ) ;
#11254=CARTESIAN_POINT ( 'NONE',  ( 61.81956123787853130, -1.983739999999999837, -1.238102447480925239 ) ) ;
#11255=DIRECTION ( 'NONE',  ( 0.8667647648559581031, 0.000000000000000000, 0.4987171968201974948 ) ) ;
#11260=DIRECTION ( 'NONE',  ( 0.9784543669157944601, 0.000000000000000000, 0.2064631973582987667 ) ) ;
#11262=LINE ( 'NONE', #9274, #19521 ) ;
#11264=CARTESIAN_POINT ( 'NONE',  ( 39.16413618835606769, 34.52875999999999834, -24.45043885672975392 ) ) ;
#11265=ORIENTED_EDGE ( 'NONE', *, *, #261, .F. ) ;
#11269=CARTESIAN_POINT ( 'NONE',  ( 59.65121809612895731, -1.983739999999999837, -2.485718937265306572 ) ) ;
#11274=CARTESIAN_POINT ( 'NONE',  ( 61.56621290189396944, -4.569743463999999200, -0.7977859469341201937 ) ) ;
#11283=DIRECTION ( 'NONE',  ( 0.000000000000000000, 1.000000000000000000, 0.000000000000000000 ) ) ;
#11294=CIRCLE ( 'NONE', #4248, 1.190625000000000488 ) ;
#11309=VECTOR ( 'NONE', #18488, 1000.000000000000000 ) ;
#11311=CARTESIAN_POINT ( 'NONE',  ( 52.65345379380397617, 38.88803500000000213, -16.29354262597895087 ) ) ;
#11312=CARTESIAN_POINT ( 'NONE',  ( 38.73829298383838449, -5.190444891651378789, -4.197541117638883712 ) ) ;
#11315=CYLINDRICAL_SURFACE ( 'NONE', #7855, 30.16249999999999076 ) ;
#11317=DIRECTION ( 'NONE',  ( 0.000000000000000000, 1.000000000000000000, 0.000000000000000000 ) ) ;
#11321=ORIENTED_EDGE ( 'NONE', *, *, #9167, .F. ) ;
#11323=DIRECTION ( 'NONE',  ( 0.05085730733808393328, 0.000000000000000000, -0.9987059298363656357 ) ) ;
#11325=EDGE_CURVE ( 'NONE', #8981, #7494, #21130, .T. ) ;
#11332=DIRECTION ( 'NONE',  ( 0.000000000000000000, 1.000000000000000000, 0.000000000000000000 ) ) ;
#11333=ORIENTED_EDGE ( 'NONE', *, *, #11498, .F. ) ;
#11335=DIRECTION ( 'NONE',  ( -0.6702301885068628895, 0.000000000000000000, -0.7421532822901579785 ) ) ;
#11343=AXIS2_PLACEMENT_3D ( 'NONE', #3068, #17990, #2846 ) ;
#11349=CYLINDRICAL_SURFACE ( 'NONE', #8940, 0.7950200000000003930 ) ;
#11353=ORIENTED_EDGE ( 'NONE', *, *, #6025, .T. ) ;
#11354=EDGE_CURVE ( 'NONE', #13139, #15569, #13083, .T. ) ;
#11362=AXIS2_PLACEMENT_3D ( 'NONE', #3216, #6538, #10276 ) ;
#11365=ORIENTED_EDGE ( 'NONE', *, *, #6053, .F. ) ;
#11367=B_SPLINE_CURVE_WITH_KNOTS ( 'NONE', 3,
 ( #20808, #5677, #2135, #8760 ),
 .UNSPECIFIED., .F., .F.,
 ( 4, 4 ),
 ( -7.968845587666753810E-05, 0.0007517777332624285547 ),
 .UNSPECIFIED. ) ;
#11368=AXIS2_PLACEMENT_3D ( 'NONE', #3978, #10721, #5743 ) ;
#11369=AXIS2_PLACEMENT_3D ( 'NONE', #19148, #909, #4014 ) ;
#11378=VERTEX_POINT ( 'NONE', #9835 ) ;
#11387=ADVANCED_FACE ( 'NONE', ( #11944 ), #112, .F. ) ;
#11389=ORIENTED_EDGE ( 'NONE', *, *, #17622, .T. ) ;
#11390=VECTOR ( 'NONE', #10579, 1000.000000000000000 ) ;
#11391=VERTEX_POINT ( 'NONE', #8622 ) ;
#11395=VECTOR ( 'NONE', #139, 1000.000000000000000 ) ;
#11407=CARTESIAN_POINT ( 'NONE',  ( 53.89155349598119926, -5.957381036604508573, -15.70768225484734160 ) ) ;
#11410=DIRECTION ( 'NONE',  ( 0.000000000000000000, 1.000000000000000000, 0.000000000000000000 ) ) ;
#11415=B_SPLINE_CURVE_WITH_KNOTS ( 'NONE', 3,
 ( #29, #8005, #21486, #14777, #1363, #15101, #11651, #6342, #18189, #19829 ),
 .UNSPECIFIED., .F., .F.,
 ( 4, 2, 2, 2, 4 ),
 ( 0.006199817995075669261, 0.006675562902873981644, 0.007151307810672294894, 0.007627052718470608145, 0.008102797626268920528 ),
 .UNSPECIFIED. ) ;
#11423=EDGE_CURVE ( 'NONE', #4193, #18443, #21142, .T. ) ;
#11425=CIRCLE ( 'NONE', #13925, 0.7950199999999982836 ) ;
#11431=CARTESIAN_POINT ( 'NONE',  ( 32.42378190387104553, 34.52875999999999834, -18.15178106273469183 ) ) ;
#11432=ADVANCED_FACE ( 'NONE', ( #19232 ), #16152, .F. ) ;
#11433=CARTESIAN_POINT ( 'NONE',  ( 30.41963056417667488, -1.983739999999999837, -8.653862521447852174 ) ) ;
#11437=CIRCLE ( 'NONE', #1889, 30.16249999999998721 ) ;
#11441=FACE_OUTER_BOUND ( 'NONE', #9007, .T. ) ;
#11447=CARTESIAN_POINT ( 'NONE',  ( 52.44708915697334106, 0.000000000000000000, 4.020247972991190188 ) ) ;
#11459=ADVANCED_FACE ( 'NONE', ( #10732 ), #2320, .T. ) ;
#11463=ORIENTED_EDGE ( 'NONE', *, *, #8438, .F. ) ;
#11465=CARTESIAN_POINT ( 'NONE',  ( 38.28489021960990613, 38.88803500000000213, 2.732679409805250703 ) ) ;
#11468=ORIENTED_EDGE ( 'NONE', *, *, #5084, .F. ) ;
#11471=CARTESIAN_POINT ( 'NONE',  ( 53.08681243026497043, 37.69777154208443193, -16.72443647847455850 ) ) ;
#11475=ORIENTED_EDGE ( 'NONE', *, *, #20311, .F. ) ;
#11481=CARTESIAN_POINT ( 'NONE',  ( 53.12465760132659653, -7.547403978437176697, -16.68255909309962348 ) ) ;
#11485=DIRECTION ( 'NONE',  ( 0.000000000000000000, 1.000000000000000000, 0.000000000000000000 ) ) ;
#11486=PLANE ( 'NONE',  #13875 ) ;
#11488=DIRECTION ( 'NONE',  ( 0.000000000000000000, -1.000000000000000000, 0.000000000000000000 ) ) ;
#11490=ORIENTED_EDGE ( 'NONE', *, *, #21118, .F. ) ;
#11498=EDGE_CURVE ( 'NONE', #19531, #7380, #15830, .T. ) ;
#11509=ORIENTED_EDGE ( 'NONE', *, *, #14253, .F. ) ;
#11515=DIRECTION ( 'NONE',  ( 0.000000000000000000, 1.000000000000000000, 0.000000000000000000 ) ) ;
#11523=DIRECTION ( 'NONE',  ( 0.000000000000000000, -1.000000000000000000, -0.000000000000000000 ) ) ;
#11527=CARTESIAN_POINT ( 'NONE',  ( 38.20361178072028707, -6.037825279267901024, -4.900284418530829633 ) ) ;
#11531=CARTESIAN_POINT ( 'NONE',  ( 42.35466991749225940, -9.531985000000000596, -17.94967221382040279 ) ) ;
#11532=CARTESIAN_POINT ( 'NONE',  ( 52.80384623828088309, 40.07865999999999929, -16.43108335029171130 ) ) ;
#11539=CARTESIAN_POINT ( 'NONE',  ( 55.33978576324753362, 34.52875999999999834, -23.05096232720518756 ) ) ;
#11540=ORIENTED_EDGE ( 'NONE', *, *, #17190, .T. ) ;
#11542=FACE_BOUND ( 'NONE', #15430, .T. ) ;
#11547=DIRECTION ( 'NONE',  ( 0.6496772031432432870, 0.000000000000000000, -0.7602101891687411683 ) ) ;
#11549=ADVANCED_FACE ( 'NONE', ( #21428 ), #9839, .T. ) ;
#11550=FACE_OUTER_BOUND ( 'NONE', #12878, .T. ) ;
#11551=PRODUCT_DEFINITION ( 'UNKNOWN', '', #17246, #826 ) ;
#11552=ORIENTED_EDGE ( 'NONE', *, *, #1009, .F. ) ;
#11555=EDGE_LOOP ( 'NONE', ( #10045, #16743, #21322, #933 ) ) ;
#11557=EDGE_CURVE ( 'NONE', #5914, #19210, #6676, .T. ) ;
#11567=DIRECTION ( 'NONE',  ( 0.05085730733808393328, 0.000000000000000000, -0.9987059298363656357 ) ) ;
#11568=EDGE_LOOP ( 'NONE', ( #15288, #841, #19740, #13684 ) ) ;
#11572=DIRECTION ( 'NONE',  ( -0.6702301885068632226, 0.000000000000000000, -0.7421532822901577564 ) ) ;
#11576=ORIENTED_EDGE ( 'NONE', *, *, #1670, .F. ) ;
#11578=EDGE_CURVE ( 'NONE', #19311, #19208, #21491, .T. ) ;
#11582=ORIENTED_EDGE ( 'NONE', *, *, #8951, .F. ) ;
#11588=CARTESIAN_POINT ( 'NONE',  ( 49.72033008250774344, 42.06303499999999929, -2.687827786179598277 ) ) ;
#11590=VECTOR ( 'NONE', #20498, 1000.000000000000114 ) ;
#11592=CARTESIAN_POINT ( 'NONE',  ( 61.56621290189396944, 0.000000000000000000, -0.7977859469341201937 ) ) ;
#11593=CARTESIAN_POINT ( 'NONE',  ( 36.80301088673436283, 0.000000000000000000, -23.10021947667301134 ) ) ;
#11597=VERTEX_POINT ( 'NONE', #2987 ) ;
#11599=LINE ( 'NONE', #18133, #5889 ) ;
#11601=EDGE_LOOP ( 'NONE', ( #5634, #12896, #16675, #19825 ) ) ;
#11602=EDGE_CURVE ( 'NONE', #21211, #10152, #667, .T. ) ;
#11608=DIRECTION ( 'NONE',  ( 0.8583349619704310207, 0.000000000000000000, -0.5130897514657826175 ) ) ;
#11609=CARTESIAN_POINT ( 'NONE',  ( 31.68988926855799448, 34.52875999999999834, 1.626235259850384418 ) ) ;
#11613=LINE ( 'NONE', #9950, #346 ) ;
#11614=EDGE_LOOP ( 'NONE', ( #2162, #16094, #21041, #15204 ) ) ;
#11619=ORIENTED_EDGE ( 'NONE', *, *, #2742, .F. ) ;
#11621=AXIS2_PLACEMENT_3D ( 'NONE', #6181, #14385, #14613 ) ;
#11625=EDGE_CURVE ( 'NONE', #5229, #16209, #10587, .T. ) ;
#11632=ORIENTED_EDGE ( 'NONE', *, *, #14653, .T. ) ;
#11636=CARTESIAN_POINT ( 'NONE',  ( 48.58367710892853353, 0.000000000000000000, -25.32442392637788231 ) ) ;
#11638=CARTESIAN_POINT ( 'NONE',  ( 52.79771328282338771, 32.54502000000000095, 3.317700572842066986 ) ) ;
#11639=CARTESIAN_POINT ( 'NONE',  ( 44.27024749654656688, 38.88803500000000213, -8.722764363618033201 ) ) ;
#11640=DIRECTION ( 'NONE',  ( 0.000000000000000000, 1.000000000000000000, 0.000000000000000000 ) ) ;
#11649=VECTOR ( 'NONE', #4905, 1000.000000000000000 ) ;
#11650=CARTESIAN_POINT ( 'NONE',  ( 57.69402548289047417, 32.54502000000000095, -20.84562559047711261 ) ) ;
#11651=CARTESIAN_POINT ( 'NONE',  ( 52.31827865322838278, 38.27710895709835626, -17.47985049647301636 ) ) ;
#11664=CARTESIAN_POINT ( 'NONE',  ( 38.96848998618624904, 40.07865999999999929, -3.934807454472129429 ) ) ;
#11670=VERTEX_POINT ( 'NONE', #8479 ) ;
#11676=ORIENTED_EDGE ( 'NONE', *, *, #11578, .F. ) ;
#11702=VECTOR ( 'NONE', #8227, 1000.000000000000000 ) ;
#11703=CARTESIAN_POINT ( 'NONE',  ( 42.35466991749225940, 42.06303499999999929, -17.94967221382040279 ) ) ;
#11704=DIRECTION ( 'NONE',  ( 0.9129422336036123742, 0.000000000000000000, -0.4080888115384289083 ) ) ;
#11706=CARTESIAN_POINT ( 'NONE',  ( 53.10651001381376091, 40.07865999999999929, -16.70269254552787075 ) ) ;
#11708=VERTEX_POINT ( 'NONE', #3412 ) ;
#11713=AXIS2_PLACEMENT_3D ( 'NONE', #7866, #11410, #1235 ) ;
#11718=VECTOR ( 'NONE', #6567, 1000.000000000000000 ) ;
#11720=CIRCLE ( 'NONE', #16994, 1.190625000000000488 ) ;
#11722=CIRCLE ( 'NONE', #1128, 0.5080000000000013394 ) ;
#11727=EDGE_CURVE ( 'NONE', #1050, #15435, #16570, .T. ) ;
#11728=CARTESIAN_POINT ( 'NONE',  ( 59.10939610998308780, 0.000000000000000000, -2.797471275456639539 ) ) ;
#11729=ORIENTED_EDGE ( 'NONE', *, *, #2511, .F. ) ;
#11732=CARTESIAN_POINT ( 'NONE',  ( 52.27672133479757832, -6.045805788883473753, -17.51606593332607176 ) ) ;
#11735=AXIS2_PLACEMENT_3D ( 'NONE', #4943, #8687, #21751 ) ;
#11755=EDGE_CURVE ( 'NONE', #20322, #10480, #6313, .T. ) ;
#11759=CARTESIAN_POINT ( 'NONE',  ( 55.33978576324753362, 34.52875999999999834, -23.05096232720518756 ) ) ;
#11760=FACE_OUTER_BOUND ( 'NONE', #12979, .T. ) ;
#11762=CARTESIAN_POINT ( 'NONE',  ( 53.84486179190094646, -76.79125307200000350, -6.412645463410259872 ) ) ;
#11764=CARTESIAN_POINT ( 'NONE',  ( 49.28028498622276032, 34.52875999999999834, -25.68670502218146368 ) ) ;
#11766=CARTESIAN_POINT ( 'NONE',  ( 44.27024749654656688, 38.88803500000000213, -8.722764363618033201 ) ) ;
#11767=AXIS2_PLACEMENT_3D ( 'NONE', #17805, #6064, #11485 ) ;
#11774=ORIENTED_EDGE ( 'NONE', *, *, #5973, .F. ) ;
#11776=CYLINDRICAL_SURFACE ( 'NONE', #20130, 9.524999999999998579 ) ;
#11778=ORIENTED_EDGE ( 'NONE', *, *, #15488, .T. ) ;
#11781=CARTESIAN_POINT ( 'NONE',  ( 38.86427657468069441, 37.69740999999999786, -4.050204114804302868 ) ) ;
#11785=SURFACE_SIDE_STYLE ('',( #21399 ) ) ;
#11790=DIRECTION ( 'NONE',  ( 0.05085730733808393328, 0.000000000000000000, -0.9987059298363656357 ) ) ;
#11791=ORIENTED_EDGE ( 'NONE', *, *, #1727, .F. ) ;
#11792=ORIENTED_EDGE ( 'NONE', *, *, #7483, .T. ) ;
#11793=CARTESIAN_POINT ( 'NONE',  ( 53.14266576735293768, -5.167590446840315543, -16.66242751532468702 ) ) ;
#11797=ORIENTED_EDGE ( 'NONE', *, *, #1514, .F. ) ;
#11805=AXIS2_PLACEMENT_3D ( 'NONE', #14605, #9703, #11255 ) ;
#11806=EDGE_CURVE ( 'NONE', #11708, #21099, #17219, .T. ) ;
#11809=DIRECTION ( 'NONE',  ( -0.1060008583745224581, 0.000000000000000000, -0.9943660382494288186 ) ) ;
#11811=CIRCLE ( 'NONE', #9686, 30.16249999999999787 ) ;
#11815=LINE ( 'NONE', #1850, #13904 ) ;
#11819=DIRECTION ( 'NONE',  ( 0.000000000000000000, 0.000000000000000000, 1.000000000000000000 ) ) ;
#11825=AXIS2_PLACEMENT_3D ( 'NONE', #17737, #17285, #7122 ) ;
#11840=CARTESIAN_POINT ( 'NONE',  ( 46.03750000000000142, -9.531985000000000596, -10.31874999999999964 ) ) ;
#11841=CARTESIAN_POINT ( 'NONE',  ( 53.54886731469894556, -5.294027063544084477, -16.17778660901759125 ) ) ;
#11845=ORIENTED_EDGE ( 'NONE', *, *, #1834, .T. ) ;
#11851=DIRECTION ( 'NONE',  ( 0.000000000000000000, -1.000000000000000000, -0.000000000000000000 ) ) ;
#11860=DIRECTION ( 'NONE',  ( 0.1060008583745224581, 0.000000000000000000, 0.9943660382494288186 ) ) ;
#11861=DIRECTION ( 'NONE',  ( 0.000000000000000000, 1.000000000000000000, 0.000000000000000000 ) ) ;
#11868=DIRECTION ( 'NONE',  ( 0.000000000000000000, -1.000000000000000000, -0.000000000000000000 ) ) ;
#11889=CARTESIAN_POINT ( 'NONE',  ( 52.44708915697334106, -1.983739999999999837, 4.020247972991190188 ) ) ;
#11896=DIRECTION ( 'NONE',  ( 0.000000000000000000, 1.000000000000000000, 0.000000000000000000 ) ) ;
#11899=CARTESIAN_POINT ( 'NONE',  ( 49.72033008250774344, -9.531985000000000596, -2.687827786179598277 ) ) ;
#11902=EDGE_CURVE ( 'NONE', #11247, #18443, #16125, .T. ) ;
#11903=CARTESIAN_POINT ( 'NONE',  ( 64.66604708500285881, 34.52875999999999834, -11.54913207920052720 ) ) ;
#11908=DIRECTION ( 'NONE',  ( -0.1060008583745200572, 0.000000000000000000, -0.9943660382494290406 ) ) ;
#11913=LINE ( 'NONE', #15142, #2227 ) ;
#11920=ORIENTED_EDGE ( 'NONE', *, *, #18355, .F. ) ;
#11925=ORIENTED_EDGE ( 'NONE', *, *, #20042, .T. ) ;
#11926=CARTESIAN_POINT ( 'NONE',  ( 42.27821610176829381, 34.52875999999999834, 7.496956594510385763 ) ) ;
#11928=ORIENTED_EDGE ( 'NONE', *, *, #21140, .F. ) ;
#11931=AXIS2_PLACEMENT_3D ( 'NONE', #1567, #6757, #342 ) ;
#11932=LINE ( 'NONE', #13291, #3669 ) ;
#11936=LINE ( 'NONE', #18666, #15117 ) ;
#11938=CARTESIAN_POINT ( 'NONE',  ( 30.97944403357121956, 0.000000000000000000, -8.103300075789407586 ) ) ;
#11941=CARTESIAN_POINT ( 'NONE',  ( 53.35716956354660567, -5.185007377690430630, -16.41558412949913404 ) ) ;
#11944=FACE_OUTER_BOUND ( 'NONE', #6041, .T. ) ;
#11947=CARTESIAN_POINT ( 'NONE',  ( 39.42154620619644589, -7.547609999999999708, -4.343957374020581241 ) ) ;
#11950=ORIENTED_EDGE ( 'NONE', *, *, #9301, .F. ) ;
#11955=ADVANCED_FACE ( 'NONE', ( #19309 ), #5602, .F. ) ;
#11960=ADVANCED_FACE ( 'NONE', ( #10704, #7702 ), #12362, .T. ) ;
#11971=EDGE_CURVE ( 'NONE', #8930, #1068, #2455, .T. ) ;
#11975=DIRECTION ( 'NONE',  ( -0.7421532822901580895, 0.000000000000000000, 0.6702301885068630005 ) ) ;
#11988=CARTESIAN_POINT ( 'NONE',  ( 52.50728002481341150, 38.88803500000000213, -18.54895932800084779 ) ) ;
#11990=ORIENTED_EDGE ( 'NONE', *, *, #21038, .T. ) ;
#11996=FACE_OUTER_BOUND ( 'NONE', #8813, .T. ) ;
#11997=EDGE_CURVE ( 'NONE', #21211, #6484, #20147, .T. ) ;
#12002=ORIENTED_EDGE ( 'NONE', *, *, #18927, .F. ) ;
#12013=PLANE ( 'NONE',  #3321 ) ;
#12016=CARTESIAN_POINT ( 'NONE',  ( 27.93207353965470574, 32.54502000000000095, -8.388685343514779902 ) ) ;
#12017=CARTESIAN_POINT ( 'NONE',  ( 42.35466991749225940, -9.531985000000000596, -17.94967221382040279 ) ) ;
#12024=CARTESIAN_POINT ( 'NONE',  ( 37.29356535768673098, -6.356984999999999886, -6.700294045292300105 ) ) ;
#12032=AXIS2_PLACEMENT_3D ( 'NONE', #7055, #21062, #10384 ) ;
#12034=CARTESIAN_POINT ( 'NONE',  ( 31.04121718565060206, 0.000000000000000000, -8.720124554639784975 ) ) ;
#12035=AXIS2_PLACEMENT_3D ( 'NONE', #16131, #7814, #14592 ) ;
#12052=CYLINDRICAL_SURFACE ( 'NONE', #18980, 0.5080000000000014504 ) ;
#12053=EDGE_CURVE ( 'NONE', #3464, #11708, #7391, .T. ) ;
#12056=CARTESIAN_POINT ( 'NONE',  ( 49.72033008250774344, 32.54502000000000095, -2.687827786179598277 ) ) ;
#12059=DIRECTION ( 'NONE',  ( 0.4987171968201936645, 0.000000000000000000, -0.8667647648559603235 ) ) ;
#12071=CARTESIAN_POINT ( 'NONE',  ( 54.55586098912687731, 32.54502000000000095, -6.056925149195119040 ) ) ;
#12074=CIRCLE ( 'NONE', #9929, 9.525000000000002132 ) ;
#12075=FACE_OUTER_BOUND ( 'NONE', #5050, .T. ) ;
#12079=CARTESIAN_POINT ( 'NONE',  ( 38.94885947252404179, -5.166721542084396823, -3.956611957468594287 ) ) ;
#12083=ADVANCED_FACE ( 'NONE', ( #2150 ), #17424, .T. ) ;
#12085=EDGE_CURVE ( 'NONE', #14379, #17300, #10997, .T. ) ;
#12100=DIRECTION ( 'NONE',  ( -0.6702301885068652210, 0.000000000000000000, -0.7421532822901560911 ) ) ;
#12102=AXIS2_PLACEMENT_3D ( 'NONE', #7032, #18863, #734 ) ;
#12105=EDGE_CURVE ( 'NONE', #13712, #3547, #10381, .T. ) ;
#12106=ADVANCED_FACE ( 'NONE', ( #713 ), #9334, .F. ) ;
#12114=CIRCLE ( 'NONE', #14954, 0.5079999999999997851 ) ;
#12125=CIRCLE ( 'NONE', #18117, 0.5079999999999996740 ) ;
#12128=ORIENTED_EDGE ( 'NONE', *, *, #36, .F. ) ;
#12131=VERTEX_POINT ( 'NONE', #18279 ) ;
#12132=EDGE_CURVE ( 'NONE', #15472, #6031, #16917, .T. ) ;
#12135=EDGE_CURVE ( 'NONE', #3524, #1698, #6947, .T. ) ;
#12140=CARTESIAN_POINT ( 'NONE',  ( 55.27198911326564001, 34.52875999999999834, 2.462719476673013830 ) ) ;
#12155=ORIENTED_EDGE ( 'NONE', *, *, #12357, .T. ) ;
#12161=EDGE_CURVE ( 'NONE', #13027, #10152, #10117, .T. ) ;
#12162=ORIENTED_EDGE ( 'NONE', *, *, #1147, .F. ) ;
#12172=DIRECTION ( 'NONE',  ( 0.000000000000000000, 1.000000000000000000, 0.000000000000000000 ) ) ;
#12173=CARTESIAN_POINT ( 'NONE',  ( 52.69120237754506064, -5.316777432816555127, -17.13598543997957080 ) ) ;
#12177=CARTESIAN_POINT ( 'NONE',  ( 54.88544852023625253, 38.88803500000000213, -18.42785536490203668 ) ) ;
#12182=CARTESIAN_POINT ( 'NONE',  ( 48.58367710892853353, 32.54502000000000095, -25.32442392637788231 ) ) ;
#12185=FACE_OUTER_BOUND ( 'NONE', #12307, .T. ) ;
#12189=CARTESIAN_POINT ( 'NONE',  ( 39.00487391863466513, 40.07742955315917044, -3.894748490060887747 ) ) ;
#12192=AXIS2_PLACEMENT_3D ( 'NONE', #6606, #16682, #6930 ) ;
#12206=CARTESIAN_POINT ( 'NONE',  ( 53.95242430215955665, 38.88803500000000213, -23.51676380836238067 ) ) ;
#12212=EDGE_CURVE ( 'NONE', #3115, #4911, #16527, .T. ) ;
#12214=LINE ( 'NONE', #10541, #2284 ) ;
#12226=EDGE_CURVE ( 'NONE', #9905, #17792, #21376, .T. ) ;
#12239=ORIENTED_EDGE ( 'NONE', *, *, #3350, .F. ) ;
#12240=CARTESIAN_POINT ( 'NONE',  ( 53.00421038040393995, 32.54502000000000095, 6.511420152579801446 ) ) ;
#12242=CARTESIAN_POINT ( 'NONE',  ( 42.79471501377724252, 32.54502000000000095, 5.049205022181460834 ) ) ;
#12247=DIRECTION ( 'NONE',  ( 0.000000000000000000, 1.000000000000000000, 0.000000000000000000 ) ) ;
#12249=EDGE_CURVE ( 'NONE', #9499, #17581, #19303, .T. ) ;
#12254=ADVANCED_FACE ( 'NONE', ( #11441 ), #13224, .F. ) ;
#12256=ADVANCED_FACE ( 'NONE', ( #11214 ), #19710, .F. ) ;
#12259=FACE_OUTER_BOUND ( 'NONE', #15595, .T. ) ;
#12263=EDGE_LOOP ( 'NONE', ( #5096, #5054, #12587, #335 ) ) ;
#12269=DIRECTION ( 'NONE',  ( 0.8583349619704310207, 0.000000000000000000, -0.5130897514657826175 ) ) ;
#12279=ORIENTED_EDGE ( 'NONE', *, *, #1833, .T. ) ;
#12281=ORIENTED_EDGE ( 'NONE', *, *, #210, .T. ) ;
#12283=CARTESIAN_POINT ( 'NONE',  ( 52.44708915697334106, -1.983739999999999837, 4.020247972991190188 ) ) ;
#12286=VERTEX_POINT ( 'NONE', #16632 ) ;
#12287=CARTESIAN_POINT ( 'NONE',  ( 46.07940063401251507, 34.52875999999999834, -26.08707253294707229 ) ) ;
#12290=DIRECTION ( 'NONE',  ( 0.6702301885068638887, 0.000000000000000000, 0.7421532822901570903 ) ) ;
#12295=CYLINDRICAL_SURFACE ( 'NONE', #17449, 0.5079999999999976756 ) ;
#12304=EDGE_CURVE ( 'NONE', #6777, #16794, #1475, .T. ) ;
#12307=EDGE_LOOP ( 'NONE', ( #14856, #6284, #11619, #20981 ) ) ;
#12311=ORIENTED_EDGE ( 'NONE', *, *, #9141, .F. ) ;
#12322=CARTESIAN_POINT ( 'NONE',  ( 51.69314645384351081, -6.356984999999999886, -17.03058447914853346 ) ) ;
#12323=CYLINDRICAL_SURFACE ( 'NONE', #1562, 30.16249999999999076 ) ;
#12327=DIRECTION ( 'NONE',  ( 0.000000000000000000, 1.000000000000000000, 0.000000000000000000 ) ) ;
#12329=ORIENTED_EDGE ( 'NONE', *, *, #12105, .T. ) ;
#12332=CARTESIAN_POINT ( 'NONE',  ( 39.11247911755811657, -5.166240873635326025, -4.078099790737317321 ) ) ;
#12333=ORIENTED_EDGE ( 'NONE', *, *, #15387, .F. ) ;
#12339=LINE ( 'NONE', #15787, #401 ) ;
#12342=CARTESIAN_POINT ( 'NONE',  ( 52.49113927203492125, -5.166360000000002728, -16.14695822742135078 ) ) ;
#12347=AXIS2_PLACEMENT_3D ( 'NONE', #4888, #3450, #18367 ) ;
#12352=EDGE_CURVE ( 'NONE', #18598, #3856, #1795, .T. ) ;
#12357=EDGE_CURVE ( 'NONE', #19608, #16034, #10836, .T. ) ;
#12359=CARTESIAN_POINT ( 'NONE',  ( 52.79771328282338771, 0.000000000000000000, 3.317700572842066986 ) ) ;
#12362=PLANE ( 'NONE',  #4569 ) ;
#12368=FACE_OUTER_BOUND ( 'NONE', #12678, .T. ) ;
#12369=ORIENTED_EDGE ( 'NONE', *, *, #5007, .F. ) ;
#12373=ORIENTED_EDGE ( 'NONE', *, *, #6584, .T. ) ;
#12381=ADVANCED_FACE ( 'NONE', ( #250 ), #6776, .T. ) ;
#12400=VERTEX_POINT ( 'NONE', #20349 ) ;
#12402=ORIENTED_EDGE ( 'NONE', *, *, #16504, .F. ) ;
#12406=DIRECTION ( 'NONE',  ( 0.000000000000000000, -1.000000000000000000, -0.000000000000000000 ) ) ;
#12411=CARTESIAN_POINT ( 'NONE',  ( 49.28028498622276032, -1.983739999999999837, -25.68670502218146368 ) ) ;
#12412=EDGE_CURVE ( 'NONE', #13623, #10463, #17480, .T. ) ;
#12422=FACE_OUTER_BOUND ( 'NONE', #10451, .T. ) ;
#12423=CIRCLE ( 'NONE', #11009, 1.190624999999997824 ) ;
#12426=ORIENTED_EDGE ( 'NONE', *, *, #1670, .T. ) ;
#12427=DIRECTION ( 'NONE',  ( -0.000000000000000000, -1.000000000000000000, 0.000000000000000000 ) ) ;
#12434=PRODUCT_CONTEXT ( 'NONE', #8467, 'mechanical' ) ;
#12439=VECTOR ( 'NONE', #17006, 1000.000000000000000 ) ;
#12454=AXIS2_PLACEMENT_3D ( 'NONE', #7887, #21368, #6224 ) ;
#12462=CARTESIAN_POINT ( 'NONE',  ( 61.83151161312219557, 32.54502000000000095, -0.3645647634491749334 ) ) ;
#12464=CARTESIAN_POINT ( 'NONE',  ( 39.82184059222445427, -6.515279778729755833, -3.101326419564407910 ) ) ;
#12467=ADVANCED_FACE ( 'NONE', ( #16157, #14496, #19235 ), #14618, .T. ) ;
#12476=CIRCLE ( 'NONE', #21285, 1.190625000000000711 ) ;
#12480=DIRECTION ( 'NONE',  ( 0.000000000000000000, 1.000000000000000000, 0.000000000000000000 ) ) ;
#12485=ORIENTED_EDGE ( 'NONE', *, *, #21422, .F. ) ;
#12489=ORIENTED_EDGE ( 'NONE', *, *, #14569, .T. ) ;
#12490=EDGE_CURVE ( 'NONE', #4928, #7839, #2659, .T. ) ;
#12497=DIRECTION ( 'NONE',  ( -0.3542738219355896501, 0.000000000000000000, -0.9351417320872542627 ) ) ;
#12503=ORIENTED_EDGE ( 'NONE', *, *, #4566, .T. ) ;
#12506=DIRECTION ( 'NONE',  ( -0.9237641507921654505, 0.000000000000000000, -0.3829618697876189803 ) ) ;
#12511=CARTESIAN_POINT ( 'NONE',  ( 46.03750000000000142, 0.000000000000000000, -10.31874999999999964 ) ) ;
#12512=CARTESIAN_POINT ( 'NONE',  ( 47.80475250345343596, 42.06303499999999929, -11.91473563638196786 ) ) ;
#12518=DIRECTION ( 'NONE',  ( -0.9987059298363657467, 0.000000000000000000, -0.05085730733808409287 ) ) ;
#12527=VECTOR ( 'NONE', #16198, 1000.000000000000114 ) ;
#12537=VERTEX_POINT ( 'NONE', #21006 ) ;
#12553=EDGE_LOOP ( 'NONE', ( #17911, #3753, #20461, #8257 ) ) ;
#12556=CARTESIAN_POINT ( 'NONE',  ( 53.84486179190094646, -76.79125307200000350, -6.412645463410259872 ) ) ;
#12563=CARTESIAN_POINT ( 'NONE',  ( 52.91086381164393515, 32.54502000000000095, 3.812938856729753301 ) ) ;
#12573=CARTESIAN_POINT ( 'NONE',  ( 39.18074928797054923, -7.516362886451771530, -3.705794944118392831 ) ) ;
#12578=EDGE_LOOP ( 'NONE', ( #7307, #20227, #12485, #19055 ) ) ;
#12579=DIRECTION ( 'NONE',  ( -0.6702301885068628895, 0.000000000000000000, -0.7421532822901579785 ) ) ;
#12581=CARTESIAN_POINT ( 'NONE',  ( 61.02111788801703085, 34.52875999999999834, -5.406220493519755088 ) ) ;
#12585=DIRECTION ( 'NONE',  ( 0.7421532822901580895, -0.000000000000000000, -0.6702301885068630005 ) ) ;
#12587=ORIENTED_EDGE ( 'NONE', *, *, #18456, .F. ) ;
#12593=ORIENTED_EDGE ( 'NONE', *, *, #8232, .F. ) ;
#12600=DIRECTION ( 'NONE',  ( 0.000000000000000000, 1.000000000000000000, 0.000000000000000000 ) ) ;
#12607=VERTEX_POINT ( 'NONE', #14390 ) ;
#12609=EDGE_CURVE ( 'NONE', #16794, #14138, #19643, .T. ) ;
#12611=VECTOR ( 'NONE', #1039, 1000.000000000000000 ) ;
#12614=CARTESIAN_POINT ( 'NONE',  ( 59.74839655170352160, -6.356984999999999886, -15.51636860603746193 ) ) ;
#12617=ORIENTED_EDGE ( 'NONE', *, *, #14926, .F. ) ;
#12618=CYLINDRICAL_SURFACE ( 'NONE', #10957, 1.190624999999997824 ) ;
#12632=CARTESIAN_POINT ( 'NONE',  ( 57.69402548289047417, 34.52875999999999834, -20.84562559047711261 ) ) ;
#12638=CARTESIAN_POINT ( 'NONE',  ( 44.27024749654614055, -6.356984999999999886, -8.722764363618502159 ) ) ;
#12642=EDGE_CURVE ( 'NONE', #10833, #13806, #11599, .T. ) ;
#12644=ORIENTED_EDGE ( 'NONE', *, *, #3397, .T. ) ;
#12652=EDGE_LOOP ( 'NONE', ( #13173, #9998, #10734, #1531, #7869 ) ) ;
#12654=ADVANCED_FACE ( 'NONE', ( #20089 ), #8058, .F. ) ;
#12657=EDGE_CURVE ( 'NONE', #17060, #17408, #15797, .T. ) ;
#12659=EDGE_CURVE ( 'NONE', #17060, #8133, #2726, .T. ) ;
#12660=CARTESIAN_POINT ( 'NONE',  ( 53.63200503474948277, -7.328454906157151783, -16.06800900404986265 ) ) ;
#12666=CARTESIAN_POINT ( 'NONE',  ( 38.94885947252404179, -5.166721542084396823, -3.956611957468594287 ) ) ;
#12673=EDGE_LOOP ( 'NONE', ( #3421, #13325, #7957 ) ) ;
#12674=( LENGTH_UNIT ( ) NAMED_UNIT ( * ) SI_UNIT ( .MILLI., .METRE. ) );
#12678=EDGE_LOOP ( 'NONE', ( #2398, #2274, #10225, #2198 ) ) ;
#12687=VECTOR ( 'NONE', #9384, 1000.000000000000000 ) ;
#12689=DIRECTION ( 'NONE',  ( -0.3542738219355860418, 0.000000000000000000, -0.9351417320872557060 ) ) ;
#12692=ORIENTED_EDGE ( 'NONE', *, *, #15112, .F. ) ;
#12698=AXIS2_PLACEMENT_3D ( 'NONE', #9843, #21574, #3018 ) ;
#12700=ORIENTED_EDGE ( 'NONE', *, *, #17880, .F. ) ;
#12703=EDGE_CURVE ( 'NONE', #21216, #1117, #21659, .T. ) ;
#12707=CARTESIAN_POINT ( 'NONE',  ( 39.93069333242032570, 38.88803500000010160, -3.008993689095761148 ) ) ;
#12711=ORIENTED_EDGE ( 'NONE', *, *, #11625, .F. ) ;
#12712=FACE_OUTER_BOUND ( 'NONE', #5819, .T. ) ;
#12717=EDGE_LOOP ( 'NONE', ( #1823, #859, #13337, #9694 ) ) ;
#12719=TOROIDAL_SURFACE ( 'NONE', #9866, 3.174999999999999822, 1.190625000000000044 ) ;
#12721=DIRECTION ( 'NONE',  ( -0.6702301885068628895, 0.000000000000000000, -0.7421532822901579785 ) ) ;
#12725=ORIENTED_EDGE ( 'NONE', *, *, #5838, .F. ) ;
#12729=AXIS2_PLACEMENT_3D ( 'NONE', #11639, #20344, #5320 ) ;
#12733=CIRCLE ( 'NONE', #20071, 1.190624999999997824 ) ;
#12739=EDGE_CURVE ( 'NONE', #10568, #12990, #7676, .T. ) ;
#12741=LINE ( 'NONE', #19021, #7561 ) ;
#12742=FACE_OUTER_BOUND ( 'NONE', #11601, .T. ) ;
#12745=CARTESIAN_POINT ( 'NONE',  ( 39.58386072796507449, 37.69740999999999786, -4.490541772578644064 ) ) ;
#12746=AXIS2_PLACEMENT_3D ( 'NONE', #9576, #1184, #7926 ) ;
#12748=CARTESIAN_POINT ( 'NONE',  ( 53.09667693522772680, 40.07859983757830946, -16.71356960103740619 ) ) ;
#12753=FACE_OUTER_BOUND ( 'NONE', #7166, .T. ) ;
#12756=VECTOR ( 'NONE', #17550, 1000.000000000000000 ) ;
#12759=VECTOR ( 'NONE', #19241, 1000.000000000000000 ) ;
#12767=CARTESIAN_POINT ( 'NONE',  ( 52.79771328282338771, 34.52875999999999834, 3.317700572842066986 ) ) ;
#12768=EDGE_CURVE ( 'NONE', #16034, #2599, #18336, .T. ) ;
#12776=CARTESIAN_POINT ( 'NONE',  ( 53.83496721834958976, -6.979221732790449551, -15.78953645305750442 ) ) ;
#12780=CIRCLE ( 'NONE', #11362, 0.7950199999999993938 ) ;
#12781=ORIENTED_EDGE ( 'NONE', *, *, #6085, .F. ) ;
#12806=DIRECTION ( 'NONE',  ( -0.9784543669157824697, 0.000000000000000000, -0.2064631973583561375 ) ) ;
#12807=AXIS2_PLACEMENT_3D ( 'NONE', #9488, #21535, #2867 ) ;
#12808=EDGE_LOOP ( 'NONE', ( #12970, #4466, #2176, #11463 ) ) ;
#12809=CYLINDRICAL_SURFACE ( 'NONE', #20946, 0.7950199999999985057 ) ;
#12810=CARTESIAN_POINT ( 'NONE',  ( 37.19264538843808765, -6.356984999999999886, -4.718486965773546871 ) ) ;
#12819=EDGE_CURVE ( 'NONE', #11144, #21347, #965, .T. ) ;
#12820=ORIENTED_EDGE ( 'NONE', *, *, #16460, .T. ) ;
#12821=EDGE_CURVE ( 'NONE', #16035, #13814, #17488, .T. ) ;
#12830=CARTESIAN_POINT ( 'NONE',  ( 39.72849559140086484, 38.13028898904873643, -3.181773261539532438 ) ) ;
#12851=AXIS2_PLACEMENT_3D ( 'NONE', #20440, #18366, #10297 ) ;
#12853=DIRECTION ( 'NONE',  ( 0.000000000000000000, -1.000000000000000000, -0.000000000000000000 ) ) ;
#12859=CARTESIAN_POINT ( 'NONE',  ( 49.13030338002142372, 109.3223030719999969, -2.154981381712871791 ) ) ;
#12866=DIRECTION ( 'NONE',  ( 0.8667647648559581031, 0.000000000000000000, 0.4987171968201974948 ) ) ;
#12869=CARTESIAN_POINT ( 'NONE',  ( 34.84490081146155660, 34.52875999999999834, -0.2108409695808725060 ) ) ;
#12878=EDGE_LOOP ( 'NONE', ( #1598, #16588, #7502, #542 ) ) ;
#12880=FACE_OUTER_BOUND ( 'NONE', #4972, .T. ) ;
#12883=AXIS2_PLACEMENT_3D ( 'NONE', #17526, #1030, #704 ) ;
#12887=CARTESIAN_POINT ( 'NONE',  ( 57.69402548289047417, 34.52875999999999834, -20.84562559047711261 ) ) ;
#12888=DIRECTION ( 'NONE',  ( 0.07875956036501312318, 0.000000000000000000, -0.9968936410927243807 ) ) ;
#12889=ADVANCED_FACE ( 'NONE', ( #5963 ), #188, .F. ) ;
#12891=DIRECTION ( 'NONE',  ( 0.9237641507921645623, 0.000000000000000000, 0.3829618697876213673 ) ) ;
#12893=DIRECTION ( 'NONE',  ( 0.000000000000000000, -1.000000000000000000, -0.000000000000000000 ) ) ;
#12895=CARTESIAN_POINT ( 'NONE',  ( 38.82016491058538321, 42.06303499999999929, -14.75770094105646812 ) ) ;
#12896=ORIENTED_EDGE ( 'NONE', *, *, #14517, .F. ) ;
#12899=CARTESIAN_POINT ( 'NONE',  ( 53.08681243026497043, 37.69777154208443193, -16.72443647847455850 ) ) ;
#12902=ADVANCED_FACE ( 'NONE', ( #8588, #13589, #20291 ), #10470, .F. ) ;
#12904=CARTESIAN_POINT ( 'NONE',  ( 43.49132289107146931, 34.52875999999999834, 4.686923926377883021 ) ) ;
#12908=CARTESIAN_POINT ( 'NONE',  ( 43.47225467835515644, -6.356984999999999886, -9.606390615345221207 ) ) ;
#12915=CARTESIAN_POINT ( 'NONE',  ( 61.83151161312219557, -1.983739999999999837, -0.3645647634491749334 ) ) ;
#12919=DIRECTION ( 'NONE',  ( 0.000000000000000000, 1.000000000000000000, 0.000000000000000000 ) ) ;
#12920=ORIENTED_EDGE ( 'NONE', *, *, #19165, .F. ) ;
#12925=CYLINDRICAL_SURFACE ( 'NONE', #12746, 0.5080000000000013394 ) ;
#12935=ORIENTED_EDGE ( 'NONE', *, *, #12412, .F. ) ;
#12937=CARTESIAN_POINT ( 'NONE',  ( 52.19198938901277529, 34.52875999999999834, 3.449560060533523487 ) ) ;
#12938=EDGE_CURVE ( 'NONE', #6597, #15472, #10698, .T. ) ;
#12940=CARTESIAN_POINT ( 'NONE',  ( 49.28028498622276032, 0.000000000000000000, -25.68670502218146368 ) ) ;
#12941=CARTESIAN_POINT ( 'NONE',  ( 36.73521423675246922, 0.000000000000000000, 2.413462327205186497 ) ) ;
#12945=EDGE_LOOP ( 'NONE', ( #13422, #14803, #2728, #4557 ) ) ;
#12946=CARTESIAN_POINT ( 'NONE',  ( 49.13030338002142372, 34.52875999999999834, -2.154981381712871791 ) ) ;
#12947=DIRECTION ( 'NONE',  ( 0.8943161143440100380, 0.000000000000000000, 0.4474356798743612806 ) ) ;
#12951=VERTEX_POINT ( 'NONE', #10366 ) ;
#12952=VERTEX_POINT ( 'NONE', #18868 ) ;
#12957=VERTEX_POINT ( 'NONE', #18753 ) ;
#12958=ORIENTED_EDGE ( 'NONE', *, *, #11727, .T. ) ;
#12965=FACE_BOUND ( 'NONE', #10405, .T. ) ;
#12970=ORIENTED_EDGE ( 'NONE', *, *, #3304, .T. ) ;
#12972=LINE ( 'NONE', #4340, #1764 ) ;
#12973=DIRECTION ( 'NONE',  ( 0.7421532822901579785, 0.000000000000000000, -0.6702301885068630005 ) ) ;
#12976=DIRECTION ( 'NONE',  ( -0.9987059298363656357, 0.000000000000000000, -0.05085730733808393328 ) ) ;
#12979=EDGE_LOOP ( 'NONE', ( #7553, #16899, #273, #11468 ) ) ;
#12990=VERTEX_POINT ( 'NONE', #409 ) ;
#12995=EDGE_CURVE ( 'NONE', #15022, #10134, #19319, .T. ) ;
#12996=CARTESIAN_POINT ( 'NONE',  ( 32.52436584422698473, 32.54502000000000095, 1.884807767196291284 ) ) ;
#13000=DIRECTION ( 'NONE',  ( 0.000000000000000000, 1.000000000000000000, 0.000000000000000000 ) ) ;
#13003=CYLINDRICAL_SURFACE ( 'NONE', #11041, 0.5080000000000005622 ) ;
#13004=DIRECTION ( 'NONE',  ( 0.000000000000000000, -1.000000000000000000, 0.000000000000000000 ) ) ;
#13012=DIRECTION ( 'NONE',  ( -0.7421532822901580895, 0.000000000000000000, 0.6702301885068630005 ) ) ;
#13017=AXIS2_PLACEMENT_3D ( 'NONE', #15179, #11851, #4882 ) ;
#13027=VERTEX_POINT ( 'NONE', #5380 ) ;
#13031=EDGE_LOOP ( 'NONE', ( #12281, #18196, #17555, #18619 ) ) ;
#13032=AXIS2_PLACEMENT_3D ( 'NONE', #9119, #14132, #15900 ) ;
#13037=EDGE_LOOP ( 'NONE', ( #16885, #16843, #4475, #14177 ) ) ;
#13039=ADVANCED_FACE ( 'NONE', ( #15250 ), #77, .F. ) ;
#13044=CARTESIAN_POINT ( 'NONE',  ( 38.23013820809905638, 32.54502000000000095, -14.22485453658974031 ) ) ;
#13051=CARTESIAN_POINT ( 'NONE',  ( 42.79471501377724252, 34.52875999999999834, 5.049205022181460834 ) ) ;
#13052=CYLINDRICAL_SURFACE ( 'NONE', #6771, 0.5079999999999996740 ) ;
#13057=EDGE_CURVE ( 'NONE', #20317, #16343, #17909, .T. ) ;
#13062=ORIENTED_EDGE ( 'NONE', *, *, #18968, .F. ) ;
#13065=AXIS2_PLACEMENT_3D ( 'NONE', #19087, #12480, #4068 ) ;
#13073=CARTESIAN_POINT ( 'NONE',  ( 30.25543876212147509, 32.54502000000000095, -19.39939755251907272 ) ) ;
#13074=CARTESIAN_POINT ( 'NONE',  ( 27.87822510359947614, 2.586003464000000029, -8.893823290944665061 ) ) ;
#13082=CARTESIAN_POINT ( 'NONE',  ( 53.25483508941461963, 34.52875999999999834, -5.879799058943532941 ) ) ;
#13083=LINE ( 'NONE', #20107, #21843 ) ;
#13085=DIRECTION ( 'NONE',  ( -0.6702301885068628895, 0.000000000000000000, -0.7421532822901579785 ) ) ;
#13087=VECTOR ( 'NONE', #1947, 1000.000000000000000 ) ;
#13093=ADVANCED_FACE ( 'NONE', ( #4065 ), #21290, .T. ) ;
#13097=CARTESIAN_POINT ( 'NONE',  ( 27.93207353965470574, -1.983739999999999837, -8.388685343514779902 ) ) ;
#13099=CIRCLE ( 'NONE', #15208, 4.365624999999999645 ) ;
#13103=FACE_OUTER_BOUND ( 'NONE', #19318, .T. ) ;
#13104=CARTESIAN_POINT ( 'NONE',  ( 38.94885947252404179, -5.166721542084396823, -3.956611957468594287 ) ) ;
#13105=DIRECTION ( 'NONE',  ( -0.4987171968201928873, 0.000000000000000000, 0.8667647648559606566 ) ) ;
#13118=DIRECTION ( 'NONE',  ( 0.000000000000000000, -1.000000000000000000, 0.000000000000000000 ) ) ;
#13119=ORIENTED_EDGE ( 'NONE', *, *, #19264, .F. ) ;
#13122=ORIENTED_EDGE ( 'NONE', *, *, #12657, .F. ) ;
#13123=B_SPLINE_CURVE_WITH_KNOTS ( 'NONE', 3,
 ( #9771, #9667, #13352, #20056, #16770 ),
 .UNSPECIFIED., .F., .F.,
 ( 4, 1, 4 ),
 ( 0.007480389903056189338, 0.007494994329912538743, 0.007509598756768888148 ),
 .UNSPECIFIED. ) ;
#13124=CARTESIAN_POINT ( 'NONE',  ( 52.91086381164393515, 34.52875999999999834, 3.812938856729753301 ) ) ;
#13128=ORIENTED_EDGE ( 'NONE', *, *, #1948, .T. ) ;
#13131=AXIS2_PLACEMENT_3D ( 'NONE', #20466, #5018, #3471 ) ;
#13132=CARTESIAN_POINT ( 'NONE',  ( 38.31330449142736683, 39.48727169022187411, -4.745061478489406959 ) ) ;
#13137=CYLINDRICAL_SURFACE ( 'NONE', #18395, 0.5080000000000010063 ) ;
#13139=VERTEX_POINT ( 'NONE', #7486 ) ;
#13141=CIRCLE ( 'NONE', #14914, 0.5080000000000014504 ) ;
#13144=FACE_OUTER_BOUND ( 'NONE', #20411, .T. ) ;
#13145=B_SPLINE_CURVE_WITH_KNOTS ( 'NONE', 3,
 ( #14410, #21125, #12748, #17836, #16180 ),
 .UNSPECIFIED., .F., .F.,
 ( 4, 1, 4 ),
 ( 0.003754349818373685799, 0.003769101685648578240, 0.003783853552923471114 ),
 .UNSPECIFIED. ) ;
#13146=ORIENTED_EDGE ( 'NONE', *, *, #10292, .F. ) ;
#13148=ORIENTED_EDGE ( 'NONE', *, *, #10606, .F. ) ;
#13149=ADVANCED_FACE ( 'NONE', ( #2727, #14255 ), #20973, .T. ) ;
#13151=ORIENTED_EDGE ( 'NONE', *, *, #6683, .F. ) ;
#13152=CARTESIAN_POINT ( 'NONE',  ( 59.65121809612895731, 34.52875999999999834, -2.485718937265306572 ) ) ;
#13160=CIRCLE ( 'NONE', #19136, 30.16250000000000497 ) ;
#13164=CARTESIAN_POINT ( 'NONE',  ( 49.72033008250774344, 42.06303499999999929, -2.687827786179598277 ) ) ;
#13167=CARTESIAN_POINT ( 'NONE',  ( 53.70970536199543233, 38.15648681541303233, -15.96454499544192096 ) ) ;
#13169=VERTEX_POINT ( 'NONE', #21071 ) ;
#13172=DIRECTION ( 'NONE',  ( 0.7421532822901579785, 0.000000000000000000, -0.6702301885068628895 ) ) ;
#13173=ORIENTED_EDGE ( 'NONE', *, *, #5550, .F. ) ;
#13175=ORIENTED_EDGE ( 'NONE', *, *, #12821, .T. ) ;
#13179=ADVANCED_FACE ( 'NONE', ( #7699, #14461, #21734 ), #16766, .T. ) ;
#13182=AXIS2_PLACEMENT_3D ( 'NONE', #12240, #10694, #4060 ) ;
#13183=CIRCLE ( 'NONE', #3637, 0.5080000000000010063 ) ;
#13200=ORIENTED_EDGE ( 'NONE', *, *, #16140, .F. ) ;
#13202=FACE_OUTER_BOUND ( 'NONE', #20697, .T. ) ;
#13208=PLANE ( 'NONE',  #9508 ) ;
#13215=DIRECTION ( 'NONE',  ( 0.000000000000000000, -1.000000000000000000, -0.000000000000000000 ) ) ;
#13224=CYLINDRICAL_SURFACE ( 'NONE', #13672, 1.190624999999999822 ) ;
#13231=CARTESIAN_POINT ( 'NONE',  ( 31.05388211198297554, 0.000000000000000000, -15.23127950648024331 ) ) ;
#13238=CIRCLE ( 'NONE', #12883, 0.5080000000000007843 ) ;
#13242=DIRECTION ( 'NONE',  ( -0.7421532822901562021, 0.000000000000000000, 0.6702301885068651099 ) ) ;
#13247=CARTESIAN_POINT ( 'NONE',  ( 46.03750000000000142, 34.52875999999999834, -10.31874999999999964 ) ) ;
#13251=FACE_OUTER_BOUND ( 'NONE', #17133, .T. ) ;
#13264=DIRECTION ( 'NONE',  ( 0.000000000000000000, -1.000000000000000000, -0.000000000000000000 ) ) ;
#13270=CYLINDRICAL_SURFACE ( 'NONE', #13981, 30.16250000000000142 ) ;
#13277=CARTESIAN_POINT ( 'NONE',  ( 53.21204579382725797, 37.69740999999999786, -16.58583161195731748 ) ) ;
#13281=DIRECTION ( 'NONE',  ( 0.000000000000000000, -1.000000000000000000, -0.000000000000000000 ) ) ;
#13288=MANIFOLD_SOLID_BREP ( 'Stock-MAS-676-1', #9572 ) ;
#13290=DIRECTION ( 'NONE',  ( 0.000000000000000000, 1.000000000000000000, 0.000000000000000000 ) ) ;
#13291=CARTESIAN_POINT ( 'NONE',  ( 59.52193197173441774, 34.52875999999999834, -3.260183413611184911 ) ) ;
#13295=ADVANCED_FACE ( 'NONE', ( #6252 ), #1605, .T. ) ;
#13300=CARTESIAN_POINT ( 'NONE',  ( 59.74839655170352160, -6.356984999999999886, -15.51636860603746193 ) ) ;
#13301=DIRECTION ( 'NONE',  ( 0.2227372614606430989, 0.000000000000000000, 0.9748785115885020280 ) ) ;
#13313=VERTEX_POINT ( 'NONE', #21506 ) ;
#13314=EDGE_CURVE ( 'NONE', #17699, #119, #6362, .T. ) ;
#13319=DIRECTION ( 'NONE',  ( -0.9724402360367336851, 0.000000000000000000, 0.2331522835762537549 ) ) ;
#13321=CARTESIAN_POINT ( 'NONE',  ( 61.65536943582333151, 34.52875999999999834, -11.98363747855214712 ) ) ;
#13325=ORIENTED_EDGE ( 'NONE', *, *, #17894, .F. ) ;
#13327=EDGE_CURVE ( 'NONE', #5503, #2509, #18945, .T. ) ;
#13328=ORIENTED_EDGE ( 'NONE', *, *, #18775, .F. ) ;
#13334=DIRECTION ( 'NONE',  ( 0.4080888115384288528, 0.000000000000000000, 0.9129422336036122632 ) ) ;
#13335=ORIENTED_EDGE ( 'NONE', *, *, #2919, .T. ) ;
#13337=ORIENTED_EDGE ( 'NONE', *, *, #18748, .F. ) ;
#13340=EDGE_CURVE ( 'NONE', #5911, #13394, #17082, .T. ) ;
#13343=ORIENTED_EDGE ( 'NONE', *, *, #20903, .T. ) ;
#13349=ORIENTED_EDGE ( 'NONE', *, *, #13660, .F. ) ;
#13352=CARTESIAN_POINT ( 'NONE',  ( 38.95864968682538176, -5.166420501038664348, -3.945715010571505310 ) ) ;
#13360=VERTEX_POINT ( 'NONE', #1927 ) ;
#13362=EDGE_LOOP ( 'NONE', ( #89, #16478, #2650, #538 ) ) ;
#13365=DIRECTION ( 'NONE',  ( -0.8583349619704310207, 0.000000000000000000, 0.5130897514657826175 ) ) ;
#13366=EDGE_LOOP ( 'NONE', ( #15282, #16377, #10263, #21173 ) ) ;
#13373=ORIENTED_EDGE ( 'NONE', *, *, #3156, .T. ) ;
#13384=ORIENTED_EDGE ( 'NONE', *, *, #12657, .T. ) ;
#13394=VERTEX_POINT ( 'NONE', #11889 ) ;
#13395=DIRECTION ( 'NONE',  ( -0.9987059298363656357, 0.000000000000000000, -0.05085730733808393328 ) ) ;
#13396=FACE_OUTER_BOUND ( 'NONE', #19971, .T. ) ;
#13398=ORIENTED_EDGE ( 'NONE', *, *, #8273, .T. ) ;
#13407=CIRCLE ( 'NONE', #8086, 30.16249999999999076 ) ;
#13409=EDGE_CURVE ( 'NONE', #17581, #13937, #1767, .T. ) ;
#13414=DIRECTION ( 'NONE',  ( 0.05085730733808393328, 0.000000000000000000, -0.9987059298363656357 ) ) ;
#13420=CIRCLE ( 'NONE', #5986, 30.16249999999998721 ) ;
#13422=ORIENTED_EDGE ( 'NONE', *, *, #13660, .T. ) ;
#13426=CARTESIAN_POINT ( 'NONE',  ( 39.47397446732132664, 38.88803500000000213, 2.793231391354656701 ) ) ;
#13432=DIRECTION ( 'NONE',  ( -0.9237641507921654505, 0.000000000000000000, -0.3829618697876189803 ) ) ;
#13436=DIRECTION ( 'NONE',  ( 0.000000000000000000, 1.000000000000000000, 0.000000000000000000 ) ) ;
#13439=AXIS2_PLACEMENT_3D ( 'NONE', #9412, #1229, #7972 ) ;
#13443=ORIENTED_EDGE ( 'NONE', *, *, #15769, .T. ) ;
#13455=DIRECTION ( 'NONE',  ( 0.000000000000000000, 1.000000000000000000, 0.000000000000000000 ) ) ;
#13456=ORIENTED_EDGE ( 'NONE', *, *, #21146, .F. ) ;
#13471=DIRECTION ( 'NONE',  ( -0.6496772031432439531, 0.000000000000000000, 0.7602101891687401691 ) ) ;
#13472=CARTESIAN_POINT ( 'NONE',  ( 52.44708915697334106, 34.52875999999999834, 4.020247972991190188 ) ) ;
#13476=DIRECTION ( 'NONE',  ( 0.3928209820863007851, 0.000000000000000000, -0.9196149607486571176 ) ) ;
#13477=CARTESIAN_POINT ( 'NONE',  ( 59.65121809612895731, -1.983739999999999837, -2.485718937265306572 ) ) ;
#13478=DIRECTION ( 'NONE',  ( 0.000000000000000000, -1.000000000000000000, 0.000000000000000000 ) ) ;
#13499=CARTESIAN_POINT ( 'NONE',  ( 49.28028498622276032, 34.52875999999999834, -25.68670502218146368 ) ) ;
#13502=DIRECTION ( 'NONE',  ( -0.4987171968201975503, 0.000000000000000000, 0.8667647648559581031 ) ) ;
#13508=CARTESIAN_POINT ( 'NONE',  ( 53.14266576735293768, -5.167590446840315543, -16.66242751532468702 ) ) ;
#13511=CIRCLE ( 'NONE', #19835, 0.5080000000000010063 ) ;
#13512=ORIENTED_EDGE ( 'NONE', *, *, #16382, .F. ) ;
#13518=ORIENTED_EDGE ( 'NONE', *, *, #15919, .F. ) ;
#13521=AXIS2_PLACEMENT_3D ( 'NONE', #12556, #4140, #10878 ) ;
#13523=CARTESIAN_POINT ( 'NONE',  ( 37.29356535768673098, -6.356984999999999886, -6.700294045292300105 ) ) ;
#13526=AXIS2_PLACEMENT_3D ( 'NONE', #1577, #14662, #19927 ) ;
#13530=CIRCLE ( 'NONE', #4359, 30.16250000000000497 ) ;
#13531=DIRECTION ( 'NONE',  ( -0.8943161143440100380, 0.000000000000000000, -0.4474356798743612806 ) ) ;
#13536=DIRECTION ( 'NONE',  ( 0.000000000000000000, 1.000000000000000000, -0.000000000000000000 ) ) ;
#13547=DIRECTION ( 'NONE',  ( 0.7421532822901569793, 0.000000000000000000, -0.6702301885068642218 ) ) ;
#13549=AXIS2_PLACEMENT_3D ( 'NONE', #5965, #6601, #15033 ) ;
#13566=VECTOR ( 'NONE', #2164, 1000.000000000000114 ) ;
#13568=VERTEX_POINT ( 'NONE', #17632 ) ;
#13575=AXIS2_PLACEMENT_3D ( 'NONE', #15495, #9044, #439 ) ;
#13576=CARTESIAN_POINT ( 'NONE',  ( 44.27024749654656688, 37.69740999999999786, -8.722764363618033201 ) ) ;
#13577=ORIENTED_EDGE ( 'NONE', *, *, #19455, .F. ) ;
#13579=DIRECTION ( 'NONE',  ( 0.000000000000000000, -1.000000000000000000, -0.000000000000000000 ) ) ;
#13582=EDGE_CURVE ( 'NONE', #19114, #8118, #5663, .T. ) ;
#13584=FACE_OUTER_BOUND ( 'NONE', #12808, .T. ) ;
#13585=CARTESIAN_POINT ( 'NONE',  ( 41.78116128337411794, 29.95901653600000003, 7.392073290253172502 ) ) ;
#13589=FACE_BOUND ( 'NONE', #20063, .T. ) ;
#13591=EDGE_CURVE ( 'NONE', #13313, #1074, #7774, .T. ) ;
#13592=DIRECTION ( 'NONE',  ( -0.3928209820863022839, 0.000000000000000000, 0.9196149607486564515 ) ) ;
#13595=CARTESIAN_POINT ( 'NONE',  ( 61.81956123787853130, 34.52875999999999834, -1.238102447480925239 ) ) ;
#13596=DIRECTION ( 'NONE',  ( 0.4080888115384288528, 0.000000000000000000, 0.9129422336036122632 ) ) ;
#13602=CARTESIAN_POINT ( 'NONE',  ( 42.92377690484065056, 0.000000000000000000, 4.437564921049077071 ) ) ;
#13611=ADVANCED_FACE ( 'NONE', ( #21154 ), #7458, .F. ) ;
#13613=EDGE_CURVE ( 'NONE', #107, #21520, #2479, .T. ) ;
#13620=DIRECTION ( 'NONE',  ( 0.6702301885068628895, 0.000000000000000000, 0.7421532822901579785 ) ) ;
#13621=CARTESIAN_POINT ( 'NONE',  ( 52.36700307908941454, -6.956221690221880749, -17.43679683612511155 ) ) ;
#13623=VERTEX_POINT ( 'NONE', #14437 ) ;
#13632=DIRECTION ( 'NONE',  ( 0.000000000000000000, -1.000000000000000000, 0.000000000000000000 ) ) ;
#13647=LINE ( 'NONE', #10194, #19081 ) ;
#13649=CARTESIAN_POINT ( 'NONE',  ( 32.52436584422698473, -1.983739999999999837, 1.884807767196291284 ) ) ;
#13653=LINE ( 'NONE', #21818, #14495 ) ;
#13660=EDGE_CURVE ( 'NONE', #18734, #17581, #7349, .T. ) ;
#13668=CARTESIAN_POINT ( 'NONE',  ( 42.94469661997857912, -76.79125307200000350, -18.48251861828712705 ) ) ;
#13671=EDGE_CURVE ( 'NONE', #1117, #16563, #2375, .T. ) ;
#13672=AXIS2_PLACEMENT_3D ( 'NONE', #4477, #18185, #13004 ) ;
#13676=ORIENTED_EDGE ( 'NONE', *, *, #20457, .F. ) ;
#13678=CARTESIAN_POINT ( 'NONE',  ( 42.66304184606194383, 32.54502000000000095, -19.22597499813143784 ) ) ;
#13684=ORIENTED_EDGE ( 'NONE', *, *, #1288, .T. ) ;
#13692=LINE ( 'NONE', #18637, #13087 ) ;
#13697=DIRECTION ( 'NONE',  ( 0.000000000000000000, 1.000000000000000000, 0.000000000000000000 ) ) ;
#13703=ORIENTED_EDGE ( 'NONE', *, *, #10758, .F. ) ;
#13712=VERTEX_POINT ( 'NONE', #19174 ) ;
#13716=ORIENTED_EDGE ( 'NONE', *, *, #12819, .T. ) ;
#13720=CARTESIAN_POINT ( 'NONE',  ( 47.80475250345343596, -6.356985000000002550, -11.91473563638196786 ) ) ;
#13724=ORIENTED_EDGE ( 'NONE', *, *, #16092, .T. ) ;
#13727=CARTESIAN_POINT ( 'NONE',  ( 56.91751438644678984, 0.000000000000000000, -20.96198986413465448 ) ) ;
#13733=EDGE_LOOP ( 'NONE', ( #21190, #6013, #20267, #14586 ) ) ;
#13748=CARTESIAN_POINT ( 'NONE',  ( 31.68988926855799448, 32.54502000000000095, 1.626235259850384418 ) ) ;
#13769=CYLINDRICAL_SURFACE ( 'NONE', #5938, 1.190624999999999378 ) ;
#13779=DIRECTION ( 'NONE',  ( 0.000000000000000000, 1.000000000000000000, 0.000000000000000000 ) ) ;
#13788=AXIS2_PLACEMENT_3D ( 'NONE', #1362, #9728, #19579 ) ;
#13794=LINE ( 'NONE', #13576, #11590 ) ;
#13797=CIRCLE ( 'NONE', #6010, 30.16249999999998721 ) ;
#13799=EDGE_LOOP ( 'NONE', ( #15813, #13512, #14414, #5695 ) ) ;
#13800=CARTESIAN_POINT ( 'NONE',  ( 38.23013820809905638, 0.000000000000000000, -14.22485453658974031 ) ) ;
#13801=FACE_OUTER_BOUND ( 'NONE', #12652, .T. ) ;
#13802=VECTOR ( 'NONE', #21477, 1000.000000000000000 ) ;
#13803=DIRECTION ( 'NONE',  ( 0.6702301885068628895, 0.000000000000000000, 0.7421532822901579785 ) ) ;
#13806=VERTEX_POINT ( 'NONE', #1470 ) ;
#13814=VERTEX_POINT ( 'NONE', #21594 ) ;
#13819=CARTESIAN_POINT ( 'NONE',  ( 59.65121809612895731, 0.000000000000000000, -2.485718937265306572 ) ) ;
#13825=AXIS2_PLACEMENT_3D ( 'NONE', #17841, #10761, #7328 ) ;
#13839=CARTESIAN_POINT ( 'NONE',  ( 53.25054008256628180, -5.160457323442601663, -16.54160408289469686 ) ) ;
#13843=EDGE_CURVE ( 'NONE', #10772, #19175, #7082, .T. ) ;
#13845=EDGE_CURVE ( 'NONE', #14616, #831, #18182, .T. ) ;
#13846=EDGE_CURVE ( 'NONE', #19005, #17300, #15224, .T. ) ;
#13850=VECTOR ( 'NONE', #12427, 1000.000000000000000 ) ;
#13851=VERTEX_POINT ( 'NONE', #8098 ) ;
#13853=AXIS2_PLACEMENT_3D ( 'NONE', #684, #14202, #16181 ) ;
#13859=CIRCLE ( 'NONE', #7113, 0.5079999999999997851 ) ;
#13869=CARTESIAN_POINT ( 'NONE',  ( 37.13209340688868565, -6.356984999999999886, -3.529402718062123689 ) ) ;
#13871=CARTESIAN_POINT ( 'NONE',  ( 42.94469661997857912, -1.983739999999999837, -18.48251861828712705 ) ) ;
#13875=AXIS2_PLACEMENT_3D ( 'NONE', #6514, #11704, #10042 ) ;
#13877=FACE_OUTER_BOUND ( 'NONE', #11555, .T. ) ;
#13878=VECTOR ( 'NONE', #7520, 1000.000000000000000 ) ;
#13879=ADVANCED_FACE ( 'NONE', ( #8418 ), #10092, .T. ) ;
#13882=DIRECTION ( 'NONE',  ( 0.5222415575336524229, 0.000000000000000000, 0.8527976052879281399 ) ) ;
#13886=VERTEX_POINT ( 'NONE', #15528 ) ;
#13887=SHAPE_DEFINITION_REPRESENTATION ( #13969, #3526 ) ;
#13892=AXIS2_PLACEMENT_3D ( 'NONE', #20458, #9987, #8748 ) ;
#13893=ORIENTED_EDGE ( 'NONE', *, *, #15112, .T. ) ;
#13897=EDGE_CURVE ( 'NONE', #7839, #17175, #3918, .T. ) ;
#13900=EDGE_CURVE ( 'NONE', #9387, #9108, #13647, .T. ) ;
#13902=ADVANCED_FACE ( 'NONE', ( #18923 ), #6770, .T. ) ;
#13904=VECTOR ( 'NONE', #8590, 1000.000000000000000 ) ;
#13911=CARTESIAN_POINT ( 'NONE',  ( 38.82016491058538321, 34.52875999999999124, -14.75770094105646812 ) ) ;
#13913=AXIS2_PLACEMENT_3D ( 'NONE', #6654, #13414, #8410 ) ;
#13916=ORIENTED_EDGE ( 'NONE', *, *, #11997, .T. ) ;
#13921=DIRECTION ( 'NONE',  ( 0.000000000000000000, -1.000000000000000000, -0.000000000000000000 ) ) ;
#13922=ORIENTED_EDGE ( 'NONE', *, *, #18198, .F. ) ;
#13923=LINE ( 'NONE', #14353, #2926 ) ;
#13925=AXIS2_PLACEMENT_3D ( 'NONE', #790, #14302, #4004 ) ;
#13927=DIRECTION ( 'NONE',  ( -0.7421532822901572013, 0.000000000000000000, 0.6702301885068637777 ) ) ;
#13928=DIRECTION ( 'NONE',  ( 0.9237641507921645623, 0.000000000000000000, 0.3829618697876213673 ) ) ;
#13930=VERTEX_POINT ( 'NONE', #20456 ) ;
#13932=FACE_OUTER_BOUND ( 'NONE', #9367, .T. ) ;
#13937=VERTEX_POINT ( 'NONE', #248 ) ;
#13944=ORIENTED_EDGE ( 'NONE', *, *, #9141, .T. ) ;
#13959=CARTESIAN_POINT ( 'NONE',  ( 61.60152099976809126, 0.000000000000000000, -12.48877542598203405 ) ) ;
#13965=FACE_OUTER_BOUND ( 'NONE', #10597, .T. ) ;
#13969=PRODUCT_DEFINITION_SHAPE ( 'NONE', 'NONE',  #11551 ) ;
#13981=AXIS2_PLACEMENT_3D ( 'NONE', #12941, #19650, #9806 ) ;
#13985=DIRECTION ( 'NONE',  ( 0.000000000000000000, 1.000000000000000000, 0.000000000000000000 ) ) ;
#13989=LINE ( 'NONE', #19365, #8147 ) ;
#13990=DIRECTION ( 'NONE',  ( -0.6702301885068630005, 0.000000000000000000, -0.7421532822901579785 ) ) ;
#13992=EDGE_LOOP ( 'NONE', ( #20217, #18012, #7405, #1485, #18209 ) ) ;
#13998=CIRCLE ( 'NONE', #7610, 0.5079999999999984528 ) ;
#14010=EDGE_CURVE ( 'NONE', #16794, #535, #14204, .T. ) ;
#14015=ORIENTED_EDGE ( 'NONE', *, *, #18691, .T. ) ;
#14017=CARTESIAN_POINT ( 'NONE',  ( 53.11256268526609858, -5.166360000000005392, -16.69599035565043366 ) ) ;
#14022=CARTESIAN_POINT ( 'NONE',  ( 0.000000000000000000, 0.000000000000000000, 0.000000000000000000 ) ) ;
#14030=VECTOR ( 'NONE', #17813, 1000.000000000000114 ) ;
#14032=CYLINDRICAL_SURFACE ( 'NONE', #19611, 0.7950199999999982836 ) ;
#14034=ORIENTED_EDGE ( 'NONE', *, *, #18725, .T. ) ;
#14044=LINE ( 'NONE', #92, #14219 ) ;
#14045=ORIENTED_EDGE ( 'NONE', *, *, #1811, .T. ) ;
#14049=ADVANCED_FACE ( 'NONE', ( #12753 ), #5545, .F. ) ;
#14054=ORIENTED_EDGE ( 'NONE', *, *, #1430, .F. ) ;
#14071=ORIENTED_EDGE ( 'NONE', *, *, #1415, .T. ) ;
#14072=ADVANCED_FACE ( 'NONE', ( #15757 ), #17504, .T. ) ;
#14078=CIRCLE ( 'NONE', #15140, 0.5080000000000023386 ) ;
#14097=LINE ( 'NONE', #17404, #2171 ) ;
#14098=ADVANCED_FACE ( 'NONE', ( #12422 ), #7653, .F. ) ;
#14104=CARTESIAN_POINT ( 'NONE',  ( 37.51913901087312553, 32.54502000000000095, -14.58057485080488114 ) ) ;
#14106=AXIS2_PLACEMENT_3D ( 'NONE', #10371, #1853, #15372 ) ;
#14113=ADVANCED_FACE ( 'NONE', ( #15648 ), #477, .F. ) ;
#14120=ORIENTED_EDGE ( 'NONE', *, *, #18672, .T. ) ;
#14121=EDGE_CURVE ( 'NONE', #21099, #13937, #13989, .T. ) ;
#14124=CARTESIAN_POINT ( 'NONE',  ( 42.66304184606194383, -9.531985000000000596, -19.22597499813143784 ) ) ;
#14126=EDGE_CURVE ( 'NONE', #17778, #4193, #5693, .T. ) ;
#14132=DIRECTION ( 'NONE',  ( -0.000000000000000000, -1.000000000000000000, 0.000000000000000000 ) ) ;
#14138=VERTEX_POINT ( 'NONE', #15856 ) ;
#14139=DIRECTION ( 'NONE',  ( 0.000000000000000000, 1.000000000000000000, 0.000000000000000000 ) ) ;
#14140=DIRECTION ( 'NONE',  ( 0.000000000000000000, 1.000000000000000000, 0.000000000000000000 ) ) ;
#14144=CARTESIAN_POINT ( 'NONE',  ( 43.29176983217143260, 37.11476346399999926, 5.154088326438659884 ) ) ;
#14151=ORIENTED_EDGE ( 'NONE', *, *, #15694, .T. ) ;
#14153=EDGE_CURVE ( 'NONE', #8481, #14418, #6035, .T. ) ;
#14155=DIRECTION ( 'NONE',  ( 0.000000000000000000, -1.000000000000000000, -0.000000000000000000 ) ) ;
#14156=ORIENTED_EDGE ( 'NONE', *, *, #16862, .F. ) ;
#14160=VERTEX_POINT ( 'NONE', #19263 ) ;
#14167=CARTESIAN_POINT ( 'NONE',  ( 46.03750000000000142, -1.983739999999999837, -10.31874999999999964 ) ) ;
#14177=ORIENTED_EDGE ( 'NONE', *, *, #11557, .F. ) ;
#14185=VERTEX_POINT ( 'NONE', #13595 ) ;
#14192=DIRECTION ( 'NONE',  ( 0.05085730733808142834, 0.000000000000000000, -0.9987059298363657467 ) ) ;
#14195=DIRECTION ( 'NONE',  ( 0.7421532822901579785, 0.000000000000000000, -0.6702301885068630005 ) ) ;
#14202=DIRECTION ( 'NONE',  ( -0.000000000000000000, -1.000000000000000000, 0.000000000000000000 ) ) ;
#14204=LINE ( 'NONE', #9307, #6405 ) ;
#14205=CIRCLE ( 'NONE', #1124, 1.190625000000000711 ) ;
#14211=VECTOR ( 'NONE', #13620, 1000.000000000000114 ) ;
#14219=VECTOR ( 'NONE', #14155, 1000.000000000000000 ) ;
#14225=EDGE_CURVE ( 'NONE', #9387, #1535, #19684, .T. ) ;
#14246=VECTOR ( 'NONE', #21047, 1000.000000000000000 ) ;
#14251=CYLINDRICAL_SURFACE ( 'NONE', #18106, 1.190625000000001155 ) ;
#14252=EDGE_CURVE ( 'NONE', #20800, #11378, #16290, .T. ) ;
#14253=EDGE_CURVE ( 'NONE', #723, #8326, #4668, .T. ) ;
#14254=LINE ( 'NONE', #5375, #9258 ) ;
#14255=FACE_BOUND ( 'NONE', #19294, .T. ) ;
#14259=DIRECTION ( 'NONE',  ( -0.9987059298363657467, 0.000000000000000000, -0.05085730733808409287 ) ) ;
#14261=ORIENTED_EDGE ( 'NONE', *, *, #15650, .F. ) ;
#14266=AXIS2_PLACEMENT_3D ( 'NONE', #9296, #7422, #9181 ) ;
#14274=EDGE_CURVE ( 'NONE', #15662, #14810, #15612, .T. ) ;
#14281=ORIENTED_EDGE ( 'NONE', *, *, #3296, .F. ) ;
#14283=CARTESIAN_POINT ( 'NONE',  ( 53.10651001381376091, 37.69740999999999786, -16.70269254552787075 ) ) ;
#14284=FACE_OUTER_BOUND ( 'NONE', #1516, .T. ) ;
#14299=VECTOR ( 'NONE', #17418, 1000.000000000000000 ) ;
#14301=EDGE_CURVE ( 'NONE', #10096, #6476, #7819, .T. ) ;
#14302=DIRECTION ( 'NONE',  ( 0.000000000000000000, 1.000000000000000000, 0.000000000000000000 ) ) ;
#14322=VERTEX_POINT ( 'NONE', #6098 ) ;
#14326=ORIENTED_EDGE ( 'NONE', *, *, #12226, .F. ) ;
#14331=CARTESIAN_POINT ( 'NONE',  ( 53.54703079237917507, -7.412034712371206702, -16.17856510773101775 ) ) ;
#14336=CARTESIAN_POINT ( 'NONE',  ( 52.97981640314721119, 40.08215061204786878, -16.84218317533225928 ) ) ;
#14341=CARTESIAN_POINT ( 'NONE',  ( 53.09665848877359196, 37.69747050103866570, -16.71358996384494233 ) ) ;
#14342=CYLINDRICAL_SURFACE ( 'NONE', #7867, 0.7950200000000003930 ) ;
#14346=PLANE ( 'NONE',  #4629 ) ;
#14347=ADVANCED_FACE ( 'NONE', ( #21865 ), #2784, .F. ) ;
#14353=CARTESIAN_POINT ( 'NONE',  ( 32.52436584422698473, -1.983739999999999837, 1.884807767196291284 ) ) ;
#14354=EDGE_CURVE ( 'NONE', #9392, #13360, #21229, .T. ) ;
#14369=EDGE_CURVE ( 'NONE', #18428, #4430, #4300, .T. ) ;
#14374=DIRECTION ( 'NONE',  ( -0.7421532822901579785, 0.000000000000000000, 0.6702301885068630005 ) ) ;
#14379=VERTEX_POINT ( 'NONE', #18645 ) ;
#14383=DIRECTION ( 'NONE',  ( 0.000000000000000000, 1.000000000000000000, 0.000000000000000000 ) ) ;
#14385=DIRECTION ( 'NONE',  ( -0.7421532822901579785, 0.000000000000000000, 0.6702301885068630005 ) ) ;
#14386=EDGE_LOOP ( 'NONE', ( #15837, #1183, #15702, #6617 ) ) ;
#14390=CARTESIAN_POINT ( 'NONE',  ( 37.51913901087312553, 0.000000000000000000, -14.58057485080488114 ) ) ;
#14391=DIRECTION ( 'NONE',  ( 0.9129422336036140395, 0.000000000000000000, -0.4080888115384250225 ) ) ;
#14410=CARTESIAN_POINT ( 'NONE',  ( 53.10651001381376091, 40.07865999999999929, -16.70269254552787075 ) ) ;
#14414=ORIENTED_EDGE ( 'NONE', *, *, #12739, .F. ) ;
#14415=DIRECTION ( 'NONE',  ( -0.9987059298363656357, 0.000000000000000000, -0.05085730733808393328 ) ) ;
#14418=VERTEX_POINT ( 'NONE', #527 ) ;
#14424=ORIENTED_EDGE ( 'NONE', *, *, #11024, .T. ) ;
#14432=LINE ( 'NONE', #18176, #9286 ) ;
#14437=CARTESIAN_POINT ( 'NONE',  ( 32.52436584422698473, -1.983739999999999837, 1.884807767196291284 ) ) ;
#14438=ORIENTED_EDGE ( 'NONE', *, *, #12212, .F. ) ;
#14441=ORIENTED_EDGE ( 'NONE', *, *, #9943, .F. ) ;
#14443=CARTESIAN_POINT ( 'NONE',  ( 53.09009400389079758, 37.69765126434668190, -16.72082518125775863 ) ) ;
#14447=DIRECTION ( 'NONE',  ( 0.7421532822901579785, 0.000000000000000000, -0.6702301885068628895 ) ) ;
#14449=FACE_OUTER_BOUND ( 'NONE', #8573, .T. ) ;
#14451=AXIS2_PLACEMENT_3D ( 'NONE', #16396, #16717, #6309 ) ;
#14452=ORIENTED_EDGE ( 'NONE', *, *, #26, .T. ) ;
#14461=FACE_BOUND ( 'NONE', #10031, .T. ) ;
#14466=ORIENTED_EDGE ( 'NONE', *, *, #6027, .F. ) ;
#14472=EDGE_CURVE ( 'NONE', #21393, #11391, #589, .T. ) ;
#14477=ORIENTED_EDGE ( 'NONE', *, *, #12105, .F. ) ;
#14480=CIRCLE ( 'NONE', #343, 0.7950199999999988387 ) ;
#14487=VERTEX_POINT ( 'NONE', #2128 ) ;
#14493=VERTEX_POINT ( 'NONE', #18930 ) ;
#14495=VECTOR ( 'NONE', #15429, 1000.000000000000114 ) ;
#14496=FACE_BOUND ( 'NONE', #9574, .T. ) ;
#14500=EDGE_LOOP ( 'NONE', ( #9243, #4715, #16293, #3090 ) ) ;
#14503=LINE ( 'NONE', #6079, #994 ) ;
#14504=AXIS2_PLACEMENT_3D ( 'NONE', #13871, #2348, #17501 ) ;
#14505=AXIS2_PLACEMENT_3D ( 'NONE', #16339, #4828, #15119 ) ;
#14511=DIRECTION ( 'NONE',  ( 0.7421532822901579785, 0.000000000000000000, -0.6702301885068630005 ) ) ;
#14513=PLANE ( 'NONE',  #1916 ) ;
#14517=EDGE_CURVE ( 'NONE', #4173, #16563, #10433, .T. ) ;
#14522=CARTESIAN_POINT ( 'NONE',  ( 53.14266576735293768, -5.167590446840315543, -16.66242751532468702 ) ) ;
#14531=CIRCLE ( 'NONE', #19777, 0.5079999999999985638 ) ;
#14535=VECTOR ( 'NONE', #21515, 1000.000000000000114 ) ;
#14536=ORIENTED_EDGE ( 'NONE', *, *, #21146, .T. ) ;
#14550=ORIENTED_EDGE ( 'NONE', *, *, #8739, .F. ) ;
#14553=DIRECTION ( 'NONE',  ( 0.000000000000000000, -1.000000000000000000, -0.000000000000000000 ) ) ;
#14554=ORIENTED_EDGE ( 'NONE', *, *, #12357, .F. ) ;
#14560=EDGE_LOOP ( 'NONE', ( #16699, #9136, #2664, #15729 ) ) ;
#14569=EDGE_CURVE ( 'NONE', #12952, #18076, #12733, .T. ) ;
#14574=ORIENTED_EDGE ( 'NONE', *, *, #12161, .F. ) ;
#14583=AXIS2_PLACEMENT_3D ( 'NONE', #9925, #2985, #14611 ) ;
#14585=DIRECTION ( 'NONE',  ( 0.7421532822901569793, 0.000000000000000000, -0.6702301885068642218 ) ) ;
#14586=ORIENTED_EDGE ( 'NONE', *, *, #19283, .F. ) ;
#14587=ORIENTED_EDGE ( 'NONE', *, *, #11971, .F. ) ;
#14590=AXIS2_PLACEMENT_3D ( 'NONE', #21320, #9489, #21209 ) ;
#14592=DIRECTION ( 'NONE',  ( 0.000000000000000000, 1.000000000000000000, 0.000000000000000000 ) ) ;
#14605=CARTESIAN_POINT ( 'NONE',  ( 59.10939610998308780, 34.52875999999999834, -2.797471275456639539 ) ) ;
#14610=CYLINDRICAL_SURFACE ( 'NONE', #16684, 30.16249999999999076 ) ;
#14611=DIRECTION ( 'NONE',  ( 0.3928209820863007851, 0.000000000000000000, -0.9196149607486571176 ) ) ;
#14613=DIRECTION ( 'NONE',  ( 0.000000000000000000, -1.000000000000000000, 0.000000000000000000 ) ) ;
#14614=CIRCLE ( 'NONE', #9275, 30.16249999999998366 ) ;
#14615=ORIENTED_EDGE ( 'NONE', *, *, #7902, .T. ) ;
#14616=VERTEX_POINT ( 'NONE', #2469 ) ;
#14618=PLANE ( 'NONE',  #7304 ) ;
#14632=CARTESIAN_POINT ( 'NONE',  ( 38.60701496492545459, 0.000000000000000000, -26.94161103631838472 ) ) ;
#14637=EDGE_LOOP ( 'NONE', ( #1304, #32, #17372, #15485 ) ) ;
#14653=EDGE_CURVE ( 'NONE', #19435, #15045, #917, .T. ) ;
#14655=DIRECTION ( 'NONE',  ( 0.9129422336036123742, 0.000000000000000000, -0.4080888115384289083 ) ) ;
#14658=CIRCLE ( 'NONE', #8977, 0.5079999999999993410 ) ;
#14662=DIRECTION ( 'NONE',  ( 0.000000000000000000, -1.000000000000000000, 0.000000000000000000 ) ) ;
#14669=CIRCLE ( 'NONE', #6168, 0.5080000000000000071 ) ;
#14671=DIRECTION ( 'NONE',  ( 0.9987059298363657467, 0.000000000000000000, 0.05085730733808445370 ) ) ;
#14677=CYLINDRICAL_SURFACE ( 'NONE', #18347, 1.190625000000000711 ) ;
#14689=CARTESIAN_POINT ( 'NONE',  ( 38.49809168999158970, 39.83951649598306233, -4.496802017747802083 ) ) ;
#14691=CIRCLE ( 'NONE', #541, 30.16250000000000497 ) ;
#14692=CARTESIAN_POINT ( 'NONE',  ( 52.50728002481341150, 38.88803500000000213, -18.54895932800084779 ) ) ;
#14694=VERTEX_POINT ( 'NONE', #11193 ) ;
#14696=EDGE_CURVE ( 'NONE', #14418, #8481, #15159, .T. ) ;
#14705=ORIENTED_EDGE ( 'NONE', *, *, #16277, .F. ) ;
#14708=ORIENTED_EDGE ( 'NONE', *, *, #5502, .F. ) ;
#14709=AXIS2_PLACEMENT_3D ( 'NONE', #12140, #15693, #10469 ) ;
#14712=CARTESIAN_POINT ( 'NONE',  ( 38.18512253410862911, -6.517595172173256124, -4.927479914652646897 ) ) ;
#14713=CARTESIAN_POINT ( 'NONE',  ( 37.13209340688868565, -6.356984999999999886, -3.529402718062123689 ) ) ;
#14714=LINE ( 'NONE', #2749, #890 ) ;
#14717=FACE_OUTER_BOUND ( 'NONE', #7597, .T. ) ;
#14721=CARTESIAN_POINT ( 'NONE',  ( 53.21069847348088189, 40.07865999999999929, -16.58732351464169597 ) ) ;
#14736=DIRECTION ( 'NONE',  ( 0.000000000000000000, 1.000000000000000000, 0.000000000000000000 ) ) ;
#14741=ORIENTED_EDGE ( 'NONE', *, *, #1033, .F. ) ;
#14744=CARTESIAN_POINT ( 'NONE',  ( 53.92488716032378449, -6.193276019600876481, -15.65869747379985988 ) ) ;
#14759=AXIS2_PLACEMENT_3D ( 'NONE', #6615, #21433, #3094 ) ;
#14760=CARTESIAN_POINT ( 'NONE',  ( 27.87822510359947614, -1.983739999999999837, -8.893823290944665061 ) ) ;
#14768=CARTESIAN_POINT ( 'NONE',  ( 52.49113927203449492, -6.356984999999999886, -16.14695822742181619 ) ) ;
#14774=EDGE_LOOP ( 'NONE', ( #4616, #14438, #12311, #2211 ) ) ;
#14776=DIRECTION ( 'NONE',  ( 0.000000000000000000, 1.000000000000000000, 0.000000000000000000 ) ) ;
#14777=CARTESIAN_POINT ( 'NONE',  ( 52.65905863606531057, 37.83483977376697993, -17.16729226877096792 ) ) ;
#14783=VERTEX_POINT ( 'NONE', #17512 ) ;
#14787=VERTEX_POINT ( 'NONE', #15981 ) ;
#14798=ADVANCED_FACE ( 'NONE', ( #4352, #1566 ), #6318, .T. ) ;
#14803=ORIENTED_EDGE ( 'NONE', *, *, #12249, .F. ) ;
#14807=DIRECTION ( 'NONE',  ( 0.000000000000000000, 1.000000000000000000, 0.000000000000000000 ) ) ;
#14810=VERTEX_POINT ( 'NONE', #9743 ) ;
#14811=ORIENTED_EDGE ( 'NONE', *, *, #18675, .T. ) ;
#14815=DIRECTION ( 'NONE',  ( 0.000000000000000000, 1.000000000000000000, 0.000000000000000000 ) ) ;
#14816=DIRECTION ( 'NONE',  ( 0.7421532822901579785, 0.000000000000000000, -0.6702301885068630005 ) ) ;
#14817=CARTESIAN_POINT ( 'NONE',  ( 30.97944403357121956, 32.54502000000000095, -8.103300075789407586 ) ) ;
#14820=ADVANCED_FACE ( 'NONE', ( #18051 ), #2909, .T. ) ;
#14822=CARTESIAN_POINT ( 'NONE',  ( 30.47347900023190803, 2.586003464000000029, -8.148724574017967015 ) ) ;
#14826=ORIENTED_EDGE ( 'NONE', *, *, #11557, .T. ) ;
#14829=DIRECTION ( 'NONE',  ( 0.000000000000000000, -1.000000000000000000, -0.000000000000000000 ) ) ;
#14839=ADVANCED_FACE ( 'NONE', ( #13202 ), #10077, .F. ) ;
#14841=CARTESIAN_POINT ( 'NONE',  ( 44.27024749654656688, -6.356984999999999886, -8.722764363618033201 ) ) ;
#14849=CARTESIAN_POINT ( 'NONE',  ( 38.82016491058538321, 0.000000000000000000, -14.75770094105646812 ) ) ;
#14854=CIRCLE ( 'NONE', #19063, 0.7950199999999982836 ) ;
#14856=ORIENTED_EDGE ( 'NONE', *, *, #1803, .T. ) ;
#14857=AXIS2_PLACEMENT_3D ( 'NONE', #10994, #17858, #2704 ) ;
#14861=CARTESIAN_POINT ( 'NONE',  ( 32.42378190387104553, -1.983739999999999837, -18.15178106273469183 ) ) ;
#14862=AXIS2_PLACEMENT_3D ( 'NONE', #17590, #17919, #11168 ) ;
#14863=CARTESIAN_POINT ( 'NONE',  ( 32.52436584422698473, 0.000000000000000000, 1.884807767196291284 ) ) ;
#14867=AXIS2_PLACEMENT_3D ( 'NONE', #6228, #6334, #12891 ) ;
#14870=DIRECTION ( 'NONE',  ( -0.2227372614607789347, 0.000000000000000000, -0.9748785115884710528 ) ) ;
#14873=DIRECTION ( 'NONE',  ( 0.2227372614607789347, 0.000000000000000000, 0.9748785115884710528 ) ) ;
#14879=CIRCLE ( 'NONE', #3208, 9.525000000000000355 ) ;
#14890=LINE ( 'NONE', #19618, #1790 ) ;
#14891=DIRECTION ( 'NONE',  ( 0.000000000000000000, -1.000000000000000000, -0.000000000000000000 ) ) ;
#14892=EDGE_LOOP ( 'NONE', ( #12781, #20080, #16987, #16224 ) ) ;
#14911=VECTOR ( 'NONE', #20135, 1000.000000000000000 ) ;
#14913=ORIENTED_EDGE ( 'NONE', *, *, #11971, .T. ) ;
#14914=AXIS2_PLACEMENT_3D ( 'NONE', #2660, #2876, #14391 ) ;
#14920=ORIENTED_EDGE ( 'NONE', *, *, #13340, .T. ) ;
#14926=EDGE_CURVE ( 'NONE', #20877, #17636, #16822, .T. ) ;
#14932=DIRECTION ( 'NONE',  ( 0.2227372614607789347, 0.000000000000000000, 0.9748785115884710528 ) ) ;
#14935=AXIS2_PLACEMENT_3D ( 'NONE', #16260, #2986, #1206 ) ;
#14937=DIRECTION ( 'NONE',  ( 0.000000000000000000, -1.000000000000000000, 0.000000000000000000 ) ) ;
#14940=CARTESIAN_POINT ( 'NONE',  ( 53.49467103128933587, 39.92874023264636207, -16.24638064876058507 ) ) ;
#14942=ORIENTED_EDGE ( 'NONE', *, *, #8042, .F. ) ;
#14945=ORIENTED_EDGE ( 'NONE', *, *, #12659, .F. ) ;
#14948=FACE_OUTER_BOUND ( 'NONE', #1650, .T. ) ;
#14954=AXIS2_PLACEMENT_3D ( 'NONE', #16996, #13697, #13592 ) ;
#14956=DIRECTION ( 'NONE',  ( 0.000000000000000000, -1.000000000000000000, -0.000000000000000000 ) ) ;
#14960=ORIENTED_EDGE ( 'NONE', *, *, #8174, .F. ) ;
#14962=DIRECTION ( 'NONE',  ( 0.8583349619704310207, 0.000000000000000000, -0.5130897514657826175 ) ) ;
#14965=ORIENTED_EDGE ( 'NONE', *, *, #5550, .T. ) ;
#14971=EDGE_CURVE ( 'NONE', #9393, #3115, #13407, .T. ) ;
#14972=EDGE_CURVE ( 'NONE', #20317, #8304, #14981, .T. ) ;
#14981=LINE ( 'NONE', #6219, #1034 ) ;
#14984=CARTESIAN_POINT ( 'NONE',  ( 32.55306802826559220, 32.54502000000000095, -17.37731658638881527 ) ) ;
#14989=LINE ( 'NONE', #21704, #9370 ) ;
#14991=AXIS2_PLACEMENT_3D ( 'NONE', #14841, #14511, #6087 ) ;
#14994=CARTESIAN_POINT ( 'NONE',  ( 43.29176983217143260, 2.586003464000000029, 5.154088326438659884 ) ) ;
#14995=DIRECTION ( 'NONE',  ( -0.8667647648559581031, 0.000000000000000000, -0.4987171968201974948 ) ) ;
#14997=EDGE_CURVE ( 'NONE', #2625, #19416, #16244, .T. ) ;
#15003=VERTEX_POINT ( 'NONE', #16512 ) ;
#15004=DIRECTION ( 'NONE',  ( 0.1060008583745199739, 0.000000000000000000, 0.9943660382494290406 ) ) ;
#15006=LINE ( 'NONE', #15107, #3844 ) ;
#15008=CARTESIAN_POINT ( 'NONE',  ( 27.40895291499714403, 34.52875999999999834, -9.088367920799473865 ) ) ;
#15021=ORIENTED_EDGE ( 'NONE', *, *, #3446, .T. ) ;
#15022=VERTEX_POINT ( 'NONE', #9428 ) ;
#15023=ADVANCED_FACE ( 'NONE', ( #9749 ), #13208, .F. ) ;
#15029=ORIENTED_EDGE ( 'NONE', *, *, #18624, .T. ) ;
#15030=ORIENTED_EDGE ( 'NONE', *, *, #1803, .F. ) ;
#15033=DIRECTION ( 'NONE',  ( 0.000000000000000000, 0.000000000000000000, 1.000000000000000000 ) ) ;
#15041=CARTESIAN_POINT ( 'NONE',  ( 53.84486179190094646, 42.06303499999999929, -6.412645463410259872 ) ) ;
#15042=CARTESIAN_POINT ( 'NONE',  ( 42.27821610176829381, 32.54502000000000095, 7.496956594510385763 ) ) ;
#15043=DIRECTION ( 'NONE',  ( -0.6702301885068630005, 0.000000000000000000, -0.7421532822901579785 ) ) ;
#15045=VERTEX_POINT ( 'NONE', #6647 ) ;
#15049=ADVANCED_FACE ( 'NONE', ( #10416 ), #5108, .T. ) ;
#15050=DIRECTION ( 'NONE',  ( -0.1060008583745224581, 0.000000000000000000, -0.9943660382494288186 ) ) ;
#15053=AXIS2_PLACEMENT_3D ( 'NONE', #11102, #8914, #12888 ) ;
#15055=CARTESIAN_POINT ( 'NONE',  ( 52.65345379380355695, 37.69740999999999786, -16.29354262597941982 ) ) ;
#15056=ORIENTED_EDGE ( 'NONE', *, *, #12352, .T. ) ;
#15065=ORIENTED_EDGE ( 'NONE', *, *, #5055, .T. ) ;
#15071=ORIENTED_EDGE ( 'NONE', *, *, #8101, .T. ) ;
#15074=EDGE_CURVE ( 'NONE', #3974, #11144, #17993, .T. ) ;
#15079=CARTESIAN_POINT ( 'NONE',  ( 39.42154620619644589, -7.547609999999999708, -4.343957374020581241 ) ) ;
#15097=LINE ( 'NONE', #13426, #14911 ) ;
#15101=CARTESIAN_POINT ( 'NONE',  ( 52.38908862829682533, 38.14157091315900061, -17.41777910622722914 ) ) ;
#15107=CARTESIAN_POINT ( 'NONE',  ( 39.11079947626275555, 32.54502000000000095, -27.65534212225540500 ) ) ;
#15112=EDGE_CURVE ( 'NONE', #4078, #1509, #17710, .T. ) ;
#15117=VECTOR ( 'NONE', #15392, 1000.000000000000000 ) ;
#15119=DIRECTION ( 'NONE',  ( 0.4987171968201974948, 0.000000000000000000, -0.8667647648559582141 ) ) ;
#15125=CARTESIAN_POINT ( 'NONE',  ( 32.17043356788648367, 34.52875999999999834, -17.71146456218788146 ) ) ;
#15127=CARTESIAN_POINT ( 'NONE',  ( 52.80360533369807285, 37.69740999999999786, -16.43086303210407451 ) ) ;
#15133=CARTESIAN_POINT ( 'NONE',  ( 44.27024749654656688, -9.531985000000000596, -8.722764363618033201 ) ) ;
#15138=CARTESIAN_POINT ( 'NONE',  ( 39.00487391863466513, 40.07742955315917044, -3.894748490060887747 ) ) ;
#15140=AXIS2_PLACEMENT_3D ( 'NONE', #7312, #15954, #12290 ) ;
#15142=CARTESIAN_POINT ( 'NONE',  ( 59.86950051480232560, -6.356984999999999886, -17.89453710146031185 ) ) ;
#15143=LINE ( 'NONE', #13164, #64 ) ;
#15144=CARTESIAN_POINT ( 'NONE',  ( 39.62791084302666178, 34.52875999999999834, -24.65774797299118859 ) ) ;
#15146=DIRECTION ( 'NONE',  ( 0.9987059298363656357, 0.000000000000000000, 0.05085730733808393328 ) ) ;
#15148=ORIENTED_EDGE ( 'NONE', *, *, #2365, .F. ) ;
#15156=VECTOR ( 'NONE', #14891, 1000.000000000000000 ) ;
#15158=LINE ( 'NONE', #13499, #18702 ) ;
#15159=CIRCLE ( 'NONE', #5612, 1.190625000000001155 ) ;
#15161=CARTESIAN_POINT ( 'NONE',  ( 46.07940063401251507, 0.000000000000000000, -26.08707253294707229 ) ) ;
#15172=AXIS2_PLACEMENT_3D ( 'NONE', #10279, #17028, #15399 ) ;
#15179=CARTESIAN_POINT ( 'NONE',  ( 48.78323016782857735, 2.586003464000000029, -25.79158832643865651 ) ) ;
#15182=LINE ( 'NONE', #5105, #6523 ) ;
#15184=CARTESIAN_POINT ( 'NONE',  ( 54.78059207134182884, -6.356984999999999886, -16.96151288338074181 ) ) ;
#15190=AXIS2_PLACEMENT_3D ( 'NONE', #7857, #1325, #1112 ) ;
#15192=DIRECTION ( 'NONE',  ( -0.7421532822901579785, 0.000000000000000000, 0.6702301885068628895 ) ) ;
#15197=DIRECTION ( 'NONE',  ( 0.000000000000000000, 1.000000000000000000, -0.000000000000000000 ) ) ;
#15204=ORIENTED_EDGE ( 'NONE', *, *, #11902, .T. ) ;
#15208=AXIS2_PLACEMENT_3D ( 'NONE', #19361, #7228, #10755 ) ;
#15224=CIRCLE ( 'NONE', #7793, 30.16249999999999076 ) ;
#15233=EDGE_CURVE ( 'NONE', #3189, #5229, #13420, .T. ) ;
#15237=ADVANCED_FACE ( 'NONE', ( #8383 ), #9945, .F. ) ;
#15240=AXIS2_PLACEMENT_3D ( 'NONE', #8031, #14807, #11572 ) ;
#15244=AXIS2_PLACEMENT_3D ( 'NONE', #11085, #804, #4016 ) ;
#15246=DIRECTION ( 'NONE',  ( 0.000000000000000000, -1.000000000000000000, -0.000000000000000000 ) ) ;
#15247=FACE_OUTER_BOUND ( 'NONE', #13366, .T. ) ;
#15250=FACE_OUTER_BOUND ( 'NONE', #9386, .T. ) ;
#15254=CARTESIAN_POINT ( 'NONE',  ( 30.50878709810603340, 34.52875999999999834, -19.83971405306587954 ) ) ;
#15257=DIRECTION ( 'NONE',  ( 0.000000000000000000, -1.000000000000000000, -0.000000000000000000 ) ) ;
#15268=EDGE_CURVE ( 'NONE', #5196, #7695, #15158, .T. ) ;
#15272=AXIS2_PLACEMENT_3D ( 'NONE', #10065, #10399, #8504 ) ;
#15273=AXIS2_PLACEMENT_3D ( 'NONE', #12034, #3750, #10483 ) ;
#15275=VECTOR ( 'NONE', #4426, 1000.000000000000000 ) ;
#15276=CARTESIAN_POINT ( 'NONE',  ( 31.02798609601340729, -1.983739999999999837, -5.485920235548950252 ) ) ;
#15277=CIRCLE ( 'NONE', #14935, 0.7950200000000003930 ) ;
#15281=DIRECTION ( 'NONE',  ( 0.000000000000000000, -1.000000000000000000, -0.000000000000000000 ) ) ;
#15282=ORIENTED_EDGE ( 'NONE', *, *, #10432, .F. ) ;
#15284=CARTESIAN_POINT ( 'NONE',  ( 32.55306802826559220, -1.983739999999999837, -17.37731658638881527 ) ) ;
#15285=CARTESIAN_POINT ( 'NONE',  ( 53.10651001381376091, -7.547610000000002373, -16.70269254552787075 ) ) ;
#15288=ORIENTED_EDGE ( 'NONE', *, *, #1811, .F. ) ;
#15292=ORIENTED_EDGE ( 'NONE', *, *, #2816, .T. ) ;
#15314=PLANE ( 'NONE',  #10326 ) ;
#15318=LINE ( 'NONE', #21713, #11718 ) ;
#15347=CARTESIAN_POINT ( 'NONE',  ( 31.68988926855799448, -1.983739999999999837, 1.626235259850384418 ) ) ;
#15356=AXIS2_PLACEMENT_3D ( 'NONE', #9319, #16410, #6112 ) ;
#15368=ORIENTED_EDGE ( 'NONE', *, *, #20746, .T. ) ;
#15369=LINE ( 'NONE', #10701, #4355 ) ;
#15372=DIRECTION ( 'NONE',  ( -0.3542738219355896501, 0.000000000000000000, -0.9351417320872542627 ) ) ;
#15374=ORIENTED_EDGE ( 'NONE', *, *, #8232, .T. ) ;
#15375=ORIENTED_EDGE ( 'NONE', *, *, #12703, .T. ) ;
#15378=DIRECTION ( 'NONE',  ( -0.9784543669157944601, 0.000000000000000000, -0.2064631973582987945 ) ) ;
#15385=LINE ( 'NONE', #4964, #17412 ) ;
#15387=EDGE_CURVE ( 'NONE', #6924, #3547, #20992, .T. ) ;
#15388=CARTESIAN_POINT ( 'NONE',  ( 27.40895291499714403, 32.54502000000000095, -9.088367920799473865 ) ) ;
#15389=CARTESIAN_POINT ( 'NONE',  ( 60.38511073144201191, 0.000000000000000000, -22.26373525985038526 ) ) ;
#15392=DIRECTION ( 'NONE',  ( 0.000000000000000000, 1.000000000000000000, 0.000000000000000000 ) ) ;
#15393=ORIENTED_EDGE ( 'NONE', *, *, #7000, .T. ) ;
#15395=PLANE ( 'NONE',  #18072 ) ;
#15396=FACE_OUTER_BOUND ( 'NONE', #18593, .T. ) ;
#15399=DIRECTION ( 'NONE',  ( -0.6496772031432439531, 0.000000000000000000, 0.7602101891687401691 ) ) ;
#15403=DIRECTION ( 'NONE',  ( -0.9129422336036514540, 0.000000000000000000, 0.4080888115383414783 ) ) ;
#15405=ORIENTED_EDGE ( 'NONE', *, *, #5180, .T. ) ;
#15425=ORIENTED_EDGE ( 'NONE', *, *, #14253, .T. ) ;
#15427=DIRECTION ( 'NONE',  ( -0.9987059298363657467, 0.000000000000000000, -0.05085730733808445370 ) ) ;
#15429=DIRECTION ( 'NONE',  ( 0.6702301885068628895, 0.000000000000000000, 0.7421532822901579785 ) ) ;
#15430=EDGE_LOOP ( 'NONE', ( #5905, #20177, #15782, #20006, #858 ) ) ;
#15435=VERTEX_POINT ( 'NONE', #13748 ) ;
#15440=EDGE_CURVE ( 'NONE', #21489, #10463, #16251, .T. ) ;
#15444=DIRECTION ( 'NONE',  ( 0.000000000000000000, -1.000000000000000000, -0.000000000000000000 ) ) ;
#15449=ORIENTED_EDGE ( 'NONE', *, *, #10762, .T. ) ;
#15453=LINE ( 'NONE', #2156, #16967 ) ;
#15454=ORIENTED_EDGE ( 'NONE', *, *, #12161, .T. ) ;
#15462=ORIENTED_EDGE ( 'NONE', *, *, #9973, .T. ) ;
#15469=FACE_OUTER_BOUND ( 'NONE', #18770, .T. ) ;
#15470=LINE ( 'NONE', #13472, #6540 ) ;
#15472=VERTEX_POINT ( 'NONE', #9297 ) ;
#15473=CARTESIAN_POINT ( 'NONE',  ( 49.28028498622276032, 0.000000000000000000, -25.68670502218146368 ) ) ;
#15474=CYLINDRICAL_SURFACE ( 'NONE', #8198, 0.5080000000000010063 ) ;
#15476=DIRECTION ( 'NONE',  ( 0.6702301885068652210, 0.000000000000000000, 0.7421532822901560911 ) ) ;
#15482=CARTESIAN_POINT ( 'NONE',  ( 30.41963056417667488, 0.000000000000000000, -8.653862521447852174 ) ) ;
#15485=ORIENTED_EDGE ( 'NONE', *, *, #12135, .F. ) ;
#15488=EDGE_CURVE ( 'NONE', #3091, #13712, #12741, .T. ) ;
#15491=ORIENTED_EDGE ( 'NONE', *, *, #1701, .T. ) ;
#15495=CARTESIAN_POINT ( 'NONE',  ( 53.84486179190094646, 0.000000000000000000, -6.412645463410259872 ) ) ;
#15496=CARTESIAN_POINT ( 'NONE',  ( 34.38097451710952868, 0.000000000000000000, 0.2081255904771098786 ) ) ;
#15502=CARTESIAN_POINT ( 'NONE',  ( 49.79678389823170903, -1.983739999999999837, -28.13445659451038594 ) ) ;
#15505=DIRECTION ( 'NONE',  ( -0.05085730733808459941, 0.000000000000000000, 0.9987059298363656357 ) ) ;
#15519=DIRECTION ( 'NONE',  ( 0.8583349619704303546, 0.000000000000000000, -0.5130897514657839498 ) ) ;
#15522=AXIS2_PLACEMENT_3D ( 'NONE', #11264, #6611, #18011 ) ;
#15525=CARTESIAN_POINT ( 'NONE',  ( 59.90456643211351917, -1.983739999999999837, -2.926035437812116946 ) ) ;
#15526=CARTESIAN_POINT ( 'NONE',  ( 39.62791084302666178, 32.54502000000000095, -24.65774797299118859 ) ) ;
#15528=CARTESIAN_POINT ( 'NONE',  ( 42.35466991749225940, -1.983739999999999837, -17.94967221382040279 ) ) ;
#15532=CARTESIAN_POINT ( 'NONE',  ( 49.13030338002142372, 42.06303499999999929, -2.154981381712871791 ) ) ;
#15534=CARTESIAN_POINT ( 'NONE',  ( 27.93207353965470574, 0.000000000000000000, -8.388685343514779902 ) ) ;
#15538=DIRECTION ( 'NONE',  ( -0.4987171968201975503, 0.000000000000000000, 0.8667647648559581031 ) ) ;
#15545=AXIS2_PLACEMENT_3D ( 'NONE', #20623, #3733, #3403 ) ;
#15559=FACE_OUTER_BOUND ( 'NONE', #20773, .T. ) ;
#15566=B_SPLINE_CURVE_WITH_KNOTS ( 'NONE', 3,
 ( #6421, #19681, #14744, #21450, #11407, #7199, #110, #20220, #11841, #11941, #13839, #13508 ),
 .UNSPECIFIED., .F., .F.,
 ( 4, 2, 2, 2, 2, 4 ),
 ( 0.003179145944081267997, 0.003422139863241870604, 0.003665133782402473211, 0.004151121620723678858, 0.004637109459044884072, 0.005123097297366089285 ),
 .UNSPECIFIED. ) ;
#15568=CARTESIAN_POINT ( 'NONE',  ( 52.19198938901277529, 0.000000000000000000, 3.449560060533523487 ) ) ;
#15569=VERTEX_POINT ( 'NONE', #14632 ) ;
#15570=CIRCLE ( 'NONE', #687, 0.5079999999999976756 ) ;
#15571=DIRECTION ( 'NONE',  ( -0.6702301885068630005, 0.000000000000000000, -0.7421532822901579785 ) ) ;
#15572=CARTESIAN_POINT ( 'NONE',  ( 43.49132289107146931, 32.54502000000000095, 4.686923926377883021 ) ) ;
#15595=EDGE_LOOP ( 'NONE', ( #20500, #2268, #19422, #10921 ) ) ;
#15601=LINE ( 'NONE', #19108, #4388 ) ;
#15606=VERTEX_POINT ( 'NONE', #6954 ) ;
#15608=DIRECTION ( 'NONE',  ( -0.3542738219355896501, 0.000000000000000000, -0.9351417320872542627 ) ) ;
#15612=CIRCLE ( 'NONE', #11713, 30.16250000000000497 ) ;
#15616=B_SPLINE_CURVE_WITH_KNOTS ( 'NONE', 3,
 ( #7536, #3672, #15743, #4108, #17386 ),
 .UNSPECIFIED., .F., .F.,
 ( 4, 1, 4 ),
 ( 0.003699823995550772550, 0.003727086906962205105, 0.003754349818373638095 ),
 .UNSPECIFIED. ) ;
#15623=VECTOR ( 'NONE', #18901, 1000.000000000000000 ) ;
#15648=FACE_OUTER_BOUND ( 'NONE', #6772, .T. ) ;
#15650=EDGE_CURVE ( 'NONE', #8830, #17565, #6149, .T. ) ;
#15653=DIRECTION ( 'NONE',  ( 0.000000000000000000, 1.000000000000000000, 0.000000000000000000 ) ) ;
#15658=AXIS2_PLACEMENT_3D ( 'NONE', #6605, #15246, #11809 ) ;
#15662=VERTEX_POINT ( 'NONE', #7190 ) ;
#15669=CIRCLE ( 'NONE', #18460, 0.7950199999999982836 ) ;
#15672=CARTESIAN_POINT ( 'NONE',  ( 42.66304184606194383, -9.531985000000000596, -19.22597499813143784 ) ) ;
#15675=EDGE_LOOP ( 'NONE', ( #10261, #8514 ) ) ;
#15678=AXIS2_PLACEMENT_3D ( 'NONE', #672, #9069, #14192 ) ;
#15684=DIRECTION ( 'NONE',  ( 0.000000000000000000, -1.000000000000000000, -0.000000000000000000 ) ) ;
#15690=FACE_OUTER_BOUND ( 'NONE', #10944, .T. ) ;
#15693=DIRECTION ( 'NONE',  ( 0.000000000000000000, 1.000000000000000000, 0.000000000000000000 ) ) ;
#15694=EDGE_CURVE ( 'NONE', #3737, #877, #5795, .T. ) ;
#15700=DIRECTION ( 'NONE',  ( 0.000000000000000000, -1.000000000000000000, -0.000000000000000000 ) ) ;
#15702=ORIENTED_EDGE ( 'NONE', *, *, #2901, .F. ) ;
#15703=ORIENTED_EDGE ( 'NONE', *, *, #9544, .T. ) ;
#15707=ORIENTED_EDGE ( 'NONE', *, *, #11055, .T. ) ;
#15715=CIRCLE ( 'NONE', #20258, 0.5079999999999996740 ) ;
#15717=DIRECTION ( 'NONE',  ( 0.7421532822901572013, 0.000000000000000000, -0.6702301885068637777 ) ) ;
#15721=EDGE_CURVE ( 'NONE', #12131, #10480, #3980, .T. ) ;
#15723=ORIENTED_EDGE ( 'NONE', *, *, #12819, .F. ) ;
#15729=ORIENTED_EDGE ( 'NONE', *, *, #17622, .F. ) ;
#15743=CARTESIAN_POINT ( 'NONE',  ( 38.98665935137078975, 37.69761546401537089, -3.914726640478982667 ) ) ;
#15757=FACE_OUTER_BOUND ( 'NONE', #4754, .T. ) ;
#15760=DIRECTION ( 'NONE',  ( -0.9943660382494290406, 0.000000000000000000, 0.1060008583745199739 ) ) ;
#15769=EDGE_CURVE ( 'NONE', #1966, #16810, #11152, .T. ) ;
#15771=ORIENTED_EDGE ( 'NONE', *, *, #4165, .F. ) ;
#15777=CARTESIAN_POINT ( 'NONE',  ( 39.62791084302666178, 34.52875999999999834, -24.65774797299118859 ) ) ;
#15779=DIRECTION ( 'NONE',  ( -0.9959941601142527912, 0.000000000000000000, -0.08941830359777887260 ) ) ;
#15782=ORIENTED_EDGE ( 'NONE', *, *, #6111, .T. ) ;
#15787=CARTESIAN_POINT ( 'NONE',  ( 61.65536943582333151, -1.983739999999999837, -11.98363747855214712 ) ) ;
#15788=ORIENTED_EDGE ( 'NONE', *, *, #12609, .F. ) ;
#15790=ORIENTED_EDGE ( 'NONE', *, *, #165, .F. ) ;
#15796=FACE_OUTER_BOUND ( 'NONE', #4309, .T. ) ;
#15797=CIRCLE ( 'NONE', #7318, 1.984375000000000000 ) ;
#15799=CARTESIAN_POINT ( 'NONE',  ( 39.07078961959606289, -4.569743463999999200, -27.14892015257980162 ) ) ;
#15807=ORIENTED_EDGE ( 'NONE', *, *, #13582, .T. ) ;
#15813=ORIENTED_EDGE ( 'NONE', *, *, #13843, .F. ) ;
#15814=AXIS2_PLACEMENT_3D ( 'NONE', #20395, #523, #5487 ) ;
#15830=LINE ( 'NONE', #2655, #12687 ) ;
#15836=ORIENTED_EDGE ( 'NONE', *, *, #20457, .T. ) ;
#15837=ORIENTED_EDGE ( 'NONE', *, *, #9724, .T. ) ;
#15840=DIRECTION ( 'NONE',  ( 0.000000000000000000, 0.000000000000000000, 1.000000000000000000 ) ) ;
#15843=ADVANCED_FACE ( 'NONE', ( #5942 ), #1301, .F. ) ;
#15853=DIRECTION ( 'NONE',  ( 0.7532174416907898573, 0.000000000000000000, 0.6577716059034334206 ) ) ;
#15856=CARTESIAN_POINT ( 'NONE',  ( 30.24348838687780727, -1.983739999999999837, -20.27293523655082552 ) ) ;
#15862=DIRECTION ( 'NONE',  ( 0.3542738219355867080, 0.000000000000000000, 0.9351417320872553729 ) ) ;
#15872=DIRECTION ( 'NONE',  ( 0.000000000000000000, 1.000000000000000000, 0.000000000000000000 ) ) ;
#15879=LINE ( 'NONE', #3926, #14246 ) ;
#15880=DIRECTION ( 'NONE',  ( -0.3542738219355896501, 0.000000000000000000, -0.9351417320872542627 ) ) ;
#15885=ORIENTED_EDGE ( 'NONE', *, *, #16755, .T. ) ;
#15889=CARTESIAN_POINT ( 'NONE',  ( 39.26944594349237150, -5.166360000000000063, -4.208320303602718582 ) ) ;
#15892=AXIS2_PLACEMENT_3D ( 'NONE', #17780, #7492, #954 ) ;
#15900=DIRECTION ( 'NONE',  ( -0.8943161143440100380, 0.000000000000000000, -0.4474356798743612806 ) ) ;
#15915=ADVANCED_FACE ( 'NONE', ( #6174 ), #1199, .T. ) ;
#15919=EDGE_CURVE ( 'NONE', #16810, #14694, #9017, .T. ) ;
#15942=VERTEX_POINT ( 'NONE', #5915 ) ;
#15947=FACE_OUTER_BOUND ( 'NONE', #5192, .T. ) ;
#15949=ORIENTED_EDGE ( 'NONE', *, *, #20068, .T. ) ;
#15954=DIRECTION ( 'NONE',  ( 0.000000000000000000, -1.000000000000000000, -0.000000000000000000 ) ) ;
#15959=AXIS2_PLACEMENT_3D ( 'NONE', #8108, #9665, #3045 ) ;
#15960=CARTESIAN_POINT ( 'NONE',  ( 38.99880687437181592, 40.07783883761410237, -3.901390339950522090 ) ) ;
#15971=DIRECTION ( 'NONE',  ( 0.000000000000000000, 1.000000000000000000, 0.000000000000000000 ) ) ;
#15981=CARTESIAN_POINT ( 'NONE',  ( 30.24348838687780727, 0.000000000000000000, -20.27293523655082552 ) ) ;
#15985=FACE_OUTER_BOUND ( 'NONE', #19687, .T. ) ;
#15988=VECTOR ( 'NONE', #20752, 1000.000000000000114 ) ;
#15995=CARTESIAN_POINT ( 'NONE',  ( 53.14266576735298031, -7.546379553159687781, -16.66242751532464084 ) ) ;
#15997=CARTESIAN_POINT ( 'NONE',  ( 55.33978576324753362, -1.983739999999999837, -23.05096232720518756 ) ) ;
#15999=EDGE_LOOP ( 'NONE', ( #15292, #17633, #14466, #5604 ) ) ;
#16003=CIRCLE ( 'NONE', #20205, 1.190625000000000488 ) ;
#16008=CYLINDRICAL_SURFACE ( 'NONE', #5993, 0.7950199999999993938 ) ;
#16009=VERTEX_POINT ( 'NONE', #3834 ) ;
#16010=DIRECTION ( 'NONE',  ( 0.9784543669157944601, -0.000000000000000000, 0.2064631973582987945 ) ) ;
#16017=ORIENTED_EDGE ( 'NONE', *, *, #9973, .F. ) ;
#16018=CARTESIAN_POINT ( 'NONE',  ( 32.18388890846549799, -4.569743463999999200, 1.507793899792891468 ) ) ;
#16021=DIRECTION ( 'NONE',  ( 0.000000000000000000, 1.000000000000000000, 0.000000000000000000 ) ) ;
#16024=VECTOR ( 'NONE', #16310, 1000.000000000000000 ) ;
#16025=ORIENTED_EDGE ( 'NONE', *, *, #19165, .T. ) ;
#16034=VERTEX_POINT ( 'NONE', #2945 ) ;
#16035=VERTEX_POINT ( 'NONE', #6473 ) ;
#16042=AXIS2_PLACEMENT_3D ( 'NONE', #18461, #14956, #6532 ) ;
#16043=CARTESIAN_POINT ( 'NONE',  ( 39.90351579496220324, 38.56174168182639761, -3.031484349533014377 ) ) ;
#16058=ORIENTED_EDGE ( 'NONE', *, *, #11354, .F. ) ;
#16062=DIRECTION ( 'NONE',  ( -0.7421532822901579785, 0.000000000000000000, 0.6702301885068628895 ) ) ;
#16073=DIRECTION ( 'NONE',  ( 0.3542738219355867080, 0.000000000000000000, 0.9351417320872553729 ) ) ;
#16076=DIRECTION ( 'NONE',  ( 0.000000000000000000, 1.000000000000000000, 0.000000000000000000 ) ) ;
#16082=DIRECTION ( 'NONE',  ( -0.8583349619704310207, 0.000000000000000000, 0.5130897514657826175 ) ) ;
#16090=DIRECTION ( 'NONE',  ( 0.000000000000000000, 1.000000000000000000, 0.000000000000000000 ) ) ;
#16091=CIRCLE ( 'NONE', #2303, 0.5079999999999984528 ) ;
#16092=EDGE_CURVE ( 'NONE', #8109, #16499, #16427, .T. ) ;
#16094=ORIENTED_EDGE ( 'NONE', *, *, #2193, .F. ) ;
#16099=DIRECTION ( 'NONE',  ( 0.000000000000000000, -1.000000000000000000, -0.000000000000000000 ) ) ;
#16103=EDGE_LOOP ( 'NONE', ( #16390, #251, #14441, #10472 ) ) ;
#16104=DIRECTION ( 'NONE',  ( -0.9129422336036127072, 0.000000000000000000, 0.4080888115384278536 ) ) ;
#16111=DIRECTION ( 'NONE',  ( 0.9959941601142464629, 0.000000000000000000, 0.08941830359784717908 ) ) ;
#16119=DIRECTION ( 'NONE',  ( 0.000000000000000000, -1.000000000000000000, -0.000000000000000000 ) ) ;
#16125=LINE ( 'NONE', #11025, #17623 ) ;
#16131=CARTESIAN_POINT ( 'NONE',  ( 44.27024749654656688, 38.88803500000000213, -8.722764363618033201 ) ) ;
#16132=ORIENTED_EDGE ( 'NONE', *, *, #21255, .F. ) ;
#16140=EDGE_CURVE ( 'NONE', #10152, #18076, #8660, .T. ) ;
#16141=EDGE_CURVE ( 'NONE', #14694, #5229, #5808, .T. ) ;
#16143=DIRECTION ( 'NONE',  ( -0.7421532822901579785, 0.000000000000000000, 0.6702301885068628895 ) ) ;
#16151=DIRECTION ( 'NONE',  ( 0.05085730733808393328, 0.000000000000000000, -0.9987059298363656357 ) ) ;
#16152=CYLINDRICAL_SURFACE ( 'NONE', #11621, 1.190625000000000711 ) ;
#16154=ORIENTED_EDGE ( 'NONE', *, *, #9761, .T. ) ;
#16156=AXIS2_PLACEMENT_3D ( 'NONE', #19934, #11110, #21480 ) ;
#16157=FACE_BOUND ( 'NONE', #18237, .T. ) ;
#16180=CARTESIAN_POINT ( 'NONE',  ( 53.08681243024872742, 40.07829845791615497, -16.72443647849243575 ) ) ;
#16181=DIRECTION ( 'NONE',  ( -0.8943161143440100380, 0.000000000000000000, -0.4474356798743612806 ) ) ;
#16183=VERTEX_POINT ( 'NONE', #15008 ) ;
#16189=EDGE_CURVE ( 'NONE', #19201, #4193, #10661, .T. ) ;
#16198=DIRECTION ( 'NONE',  ( 0.7421532822901579785, 0.000000000000000000, -0.6702301885068628895 ) ) ;
#16199=CARTESIAN_POINT ( 'NONE',  ( 42.92377690484065056, 34.52875999999999834, 4.437564921049077071 ) ) ;
#16205=CARTESIAN_POINT ( 'NONE',  ( 36.73521423675246922, 34.52875999999999834, 2.413462327205186497 ) ) ;
#16209=VERTEX_POINT ( 'NONE', #5794 ) ;
#16210=FACE_OUTER_BOUND ( 'NONE', #21842, .T. ) ;
#16211=DIRECTION ( 'NONE',  ( 0.000000000000000000, -1.000000000000000000, 0.000000000000000000 ) ) ;
#16213=EDGE_CURVE ( 'NONE', #18152, #12400, #7935, .T. ) ;
#16215=DIRECTION ( 'NONE',  ( 0.7421532822901579785, 0.000000000000000000, -0.6702301885068628895 ) ) ;
#16221=CARTESIAN_POINT ( 'NONE',  ( 31.05388211198297554, 32.54502000000000095, -15.23127950648024331 ) ) ;
#16224=ORIENTED_EDGE ( 'NONE', *, *, #18333, .F. ) ;
#16230=DIRECTION ( 'NONE',  ( 0.000000000000000000, -1.000000000000000000, 0.000000000000000000 ) ) ;
#16233=DIRECTION ( 'NONE',  ( -0.000000000000000000, -1.000000000000000000, 0.000000000000000000 ) ) ;
#16241=CARTESIAN_POINT ( 'NONE',  ( 32.52436584422698473, 32.54502000000000095, 1.884807767196291284 ) ) ;
#16244=CIRCLE ( 'NONE', #19035, 0.5079999999999965654 ) ;
#16247=ORIENTED_EDGE ( 'NONE', *, *, #2025, .T. ) ;
#16250=FACE_OUTER_BOUND ( 'NONE', #11154, .T. ) ;
#16251=CIRCLE ( 'NONE', #21879, 0.5079999999999984528 ) ;
#16256=ORIENTED_EDGE ( 'NONE', *, *, #18456, .T. ) ;
#16260=CARTESIAN_POINT ( 'NONE',  ( 42.94469661997857912, 32.54502000000000095, -18.48251861828712705 ) ) ;
#16273=FACE_OUTER_BOUND ( 'NONE', #6369, .T. ) ;
#16275=AXIS2_PLACEMENT_3D ( 'NONE', #19787, #18038, #11183 ) ;
#16277=EDGE_CURVE ( 'NONE', #10812, #5142, #11367, .T. ) ;
#16282=ORIENTED_EDGE ( 'NONE', *, *, #3410, .T. ) ;
#16286=DIRECTION ( 'NONE',  ( 0.9987059298363656357, 0.000000000000000000, 0.05085730733808393328 ) ) ;
#16288=AXIS2_PLACEMENT_3D ( 'NONE', #10426, #18815, #20576 ) ;
#16290=LINE ( 'NONE', #17939, #4993 ) ;
#16293=ORIENTED_EDGE ( 'NONE', *, *, #1033, .T. ) ;
#16303=PLANE ( 'NONE',  #20621 ) ;
#16310=DIRECTION ( 'NONE',  ( 0.000000000000000000, 1.000000000000000000, 0.000000000000000000 ) ) ;
#16321=FACE_OUTER_BOUND ( 'NONE', #14892, .T. ) ;
#16324=ORIENTED_EDGE ( 'NONE', *, *, #18198, .T. ) ;
#16327=AXIS2_PLACEMENT_3D ( 'NONE', #3541, #18784, #10277 ) ;
#16329=ORIENTED_EDGE ( 'NONE', *, *, #11902, .F. ) ;
#16339=CARTESIAN_POINT ( 'NONE',  ( 45.99559936598748777, 0.000000000000000000, 5.449572532947073000 ) ) ;
#16343=VERTEX_POINT ( 'NONE', #10872 ) ;
#16346=AXIS2_PLACEMENT_3D ( 'NONE', #10987, #20599, #5457 ) ;
#16348=CARTESIAN_POINT ( 'NONE',  ( 47.80475250345343596, 40.07865999999999929, -11.91473563638196786 ) ) ;
#16349=ORIENTED_EDGE ( 'NONE', *, *, #21331, .T. ) ;
#16355=ADVANCED_FACE ( 'NONE', ( #15985 ), #18935, .F. ) ;
#16365=DIRECTION ( 'NONE',  ( 0.000000000000000000, -1.000000000000000000, 0.000000000000000000 ) ) ;
#16368=CARTESIAN_POINT ( 'NONE',  ( 53.31385684162800942, 37.72911631579626146, -16.46698546251109008 ) ) ;
#16374=DIRECTION ( 'NONE',  ( 0.000000000000000000, 1.000000000000000000, 0.000000000000000000 ) ) ;
#16377=ORIENTED_EDGE ( 'NONE', *, *, #7611, .F. ) ;
#16382=EDGE_CURVE ( 'NONE', #12990, #10772, #12214, .T. ) ;
#16390=ORIENTED_EDGE ( 'NONE', *, *, #16436, .F. ) ;
#16396=CARTESIAN_POINT ( 'NONE',  ( 61.56621290189396944, 32.54502000000000095, -0.7977859469341201937 ) ) ;
#16398=CARTESIAN_POINT ( 'NONE',  ( 32.10373694497760511, -6.356984999999999886, -3.785462747693984831 ) ) ;
#16410=DIRECTION ( 'NONE',  ( 0.000000000000000000, -1.000000000000000000, -0.000000000000000000 ) ) ;
#16411=VECTOR ( 'NONE', #1915, 1000.000000000000000 ) ;
#16421=CARTESIAN_POINT ( 'NONE',  ( 61.03378281434940078, 0.000000000000000000, -11.91737544536021431 ) ) ;
#16422=DIRECTION ( 'NONE',  ( 0.7421532822901579785, 0.000000000000000000, -0.6702301885068628895 ) ) ;
#16427=CIRCLE ( 'NONE', #8985, 0.5080000000000022276 ) ;
#16428=DIRECTION ( 'NONE',  ( 0.6702301885068638887, 0.000000000000000000, 0.7421532822901570903 ) ) ;
#16434=DIRECTION ( 'NONE',  ( -0.7421532822901579785, 0.000000000000000000, 0.6702301885068630005 ) ) ;
#16436=EDGE_CURVE ( 'NONE', #13360, #14322, #14669, .T. ) ;
#16453=ORIENTED_EDGE ( 'NONE', *, *, #1816, .T. ) ;
#16454=EDGE_LOOP ( 'NONE', ( #15836, #7047, #13577, #20705 ) ) ;
#16460=EDGE_CURVE ( 'NONE', #16563, #17300, #7575, .T. ) ;
#16461=ORIENTED_EDGE ( 'NONE', *, *, #11755, .T. ) ;
#16462=EDGE_CURVE ( 'NONE', #16972, #14185, #19599, .T. ) ;
#16467=LINE ( 'NONE', #8041, #9586 ) ;
#16468=CYLINDRICAL_SURFACE ( 'NONE', #19218, 1.190625000000000711 ) ;
#16470=CARTESIAN_POINT ( 'NONE',  ( 27.93207353965470574, 0.000000000000000000, -8.388685343514779902 ) ) ;
#16476=CARTESIAN_POINT ( 'NONE',  ( 50.52547294529469468, 38.88803500000000213, -18.64987929725020521 ) ) ;
#16477=ORIENTED_EDGE ( 'NONE', *, *, #16462, .F. ) ;
#16478=ORIENTED_EDGE ( 'NONE', *, *, #6855, .F. ) ;
#16480=CARTESIAN_POINT ( 'NONE',  ( 30.41963056417667488, 0.000000000000000000, -8.653862521447852174 ) ) ;
#16499=VERTEX_POINT ( 'NONE', #12767 ) ;
#16504=EDGE_CURVE ( 'NONE', #9951, #1425, #7987, .T. ) ;
#16512=CARTESIAN_POINT ( 'NONE',  ( 53.25483508941461963, -1.983739999999997838, -5.879799058943532941 ) ) ;
#16524=ORIENTED_EDGE ( 'NONE', *, *, #9775, .F. ) ;
#16527=LINE ( 'NONE', #1358, #12611 ) ;
#16544=ORIENTED_EDGE ( 'NONE', *, *, #8406, .F. ) ;
#16549=EDGE_CURVE ( 'NONE', #16977, #1209, #2992, .T. ) ;
#16556=ORIENTED_EDGE ( 'NONE', *, *, #3350, .T. ) ;
#16557=ORIENTED_EDGE ( 'NONE', *, *, #15721, .T. ) ;
#16560=ADVANCED_FACE ( 'NONE', ( #12880 ), #16303, .F. ) ;
#16562=CARTESIAN_POINT ( 'NONE',  ( 61.81956123787853130, 32.54502000000000095, -1.238102447480925239 ) ) ;
#16563=VERTEX_POINT ( 'NONE', #13097 ) ;
#16567=DIRECTION ( 'NONE',  ( -0.7532174416907914116, 0.000000000000000000, -0.6577716059034314222 ) ) ;
#16570=CIRCLE ( 'NONE', #4910, 0.5080000000000013394 ) ;
#16571=B_SPLINE_CURVE_WITH_KNOTS ( 'NONE', 3,
 ( #7587, #17872, #11007, #11120, #19188, #21063, #4158, #2497, #4054, #12464, #7690, #10797, #17766, #5913, #5818, #12573, #9451, #17542 ),
 .UNSPECIFIED., .F., .F.,
 ( 4, 2, 2, 2, 2, 2, 2, 2, 4 ),
 ( 0.000000000000000000, 0.0004692937272967113212, 0.0009385874545934226425, 0.001407881181890133964, 0.001877174909186845285, 0.002346468636483556823, 0.002815762363780267927, 0.003285056091076979032, 0.003754349818373690570 ),
 .UNSPECIFIED. ) ;
#16572=DIRECTION ( 'NONE',  ( 0.000000000000000000, -1.000000000000000000, -0.000000000000000000 ) ) ;
#16575=DIRECTION ( 'NONE',  ( -0.9987059298363657467, 0.000000000000000000, -0.05085730733808409287 ) ) ;
#16577=EDGE_CURVE ( 'NONE', #1966, #10716, #15182, .T. ) ;
#16580=CARTESIAN_POINT ( 'NONE',  ( 57.35354854712898742, 37.11476346399999926, -21.22263945788050776 ) ) ;
#16583=CARTESIAN_POINT ( 'NONE',  ( 53.84899360340892827, 39.04632977872977051, -15.76908876899390322 ) ) ;
#16588=ORIENTED_EDGE ( 'NONE', *, *, #17494, .F. ) ;
#16594=AXIS2_PLACEMENT_3D ( 'NONE', #17018, #101, #3326 ) ;
#16599=CARTESIAN_POINT ( 'NONE',  ( 39.62791084302666178, 34.52875999999999834, -24.65774797299118859 ) ) ;
#16613=CARTESIAN_POINT ( 'NONE',  ( 45.99559936598748777, 34.52875999999999834, 5.449572532947073000 ) ) ;
#16619=CIRCLE ( 'NONE', #3180, 0.7950200000000003930 ) ;
#16623=DIRECTION ( 'NONE',  ( -0.7421532822901579785, 0.000000000000000000, 0.6702301885068628895 ) ) ;
#16630=CARTESIAN_POINT ( 'NONE',  ( 35.15748561355322011, 34.52875999999999834, 0.3244898641346534163 ) ) ;
#16632=CARTESIAN_POINT ( 'NONE',  ( 39.00487391863466513, 40.07742955315917044, -3.894748490060887747 ) ) ;
#16637=CARTESIAN_POINT ( 'NONE',  ( 34.72145145287101542, 34.52875999999999834, 0.5851394578805096947 ) ) ;
#16645=ORIENTED_EDGE ( 'NONE', *, *, #9399, .F. ) ;
#16653=AXIS2_PLACEMENT_3D ( 'NONE', #16398, #12976, #7976 ) ;
#16655=PRESENTATION_STYLE_ASSIGNMENT (( #9682 ) ) ;
#16660=ORIENTED_EDGE ( 'NONE', *, *, #19653, .T. ) ;
#16670=ORIENTED_EDGE ( 'NONE', *, *, #9544, .F. ) ;
#16674=CARTESIAN_POINT ( 'NONE',  ( 39.73003449695463019, 38.88803500000000213, -2.235125070556357674 ) ) ;
#16675=ORIENTED_EDGE ( 'NONE', *, *, #5574, .F. ) ;
#16682=DIRECTION ( 'NONE',  ( 0.000000000000000000, 1.000000000000000000, 0.000000000000000000 ) ) ;
#16684=AXIS2_PLACEMENT_3D ( 'NONE', #4195, #21318, #11260 ) ;
#16691=ORIENTED_EDGE ( 'NONE', *, *, #1258, .F. ) ;
#16692=ORIENTED_EDGE ( 'NONE', *, *, #2600, .T. ) ;
#16694=DIRECTION ( 'NONE',  ( 0.000000000000000000, -1.000000000000000000, 0.000000000000000000 ) ) ;
#16697=ORIENTED_EDGE ( 'NONE', *, *, #20701, .F. ) ;
#16699=ORIENTED_EDGE ( 'NONE', *, *, #10606, .T. ) ;
#16709=FACE_OUTER_BOUND ( 'NONE', #6264, .T. ) ;
#16716=DIRECTION ( 'NONE',  ( -0.7421532822901572013, 0.000000000000000000, 0.6702301885068637777 ) ) ;
#16717=DIRECTION ( 'NONE',  ( 0.000000000000000000, -1.000000000000000000, -0.000000000000000000 ) ) ;
#16725=LINE ( 'NONE', #18798, #9468 ) ;
#16730=VERTEX_POINT ( 'NONE', #18265 ) ;
#16743=ORIENTED_EDGE ( 'NONE', *, *, #286, .T. ) ;
#16748=DIRECTION ( 'NONE',  ( 0.000000000000000000, 1.000000000000000000, 0.000000000000000000 ) ) ;
#16749=CARTESIAN_POINT ( 'NONE',  ( 61.09555596642878328, -1.983739999999999837, -12.53419992421059348 ) ) ;
#16752=AXIS2_PLACEMENT_3D ( 'NONE', #2424, #20763, #2084 ) ;
#16753=ORIENTED_EDGE ( 'NONE', *, *, #1258, .T. ) ;
#16755=EDGE_CURVE ( 'NONE', #11247, #9392, #17429, .T. ) ;
#16762=CARTESIAN_POINT ( 'NONE',  ( 38.24361653725164700, 38.57685578888346356, -4.842928593324986153 ) ) ;
#16766=PLANE ( 'NONE',  #8721 ) ;
#16770=CARTESIAN_POINT ( 'NONE',  ( 38.96848998618624904, -5.166360000000000063, -3.934807454472129429 ) ) ;
#16781=DIRECTION ( 'NONE',  ( -0.000000000000000000, -1.000000000000000000, 0.000000000000000000 ) ) ;
#16783=CIRCLE ( 'NONE', #12192, 0.5079999999999984528 ) ;
#16786=DIRECTION ( 'NONE',  ( 0.4080888115384288528, 0.000000000000000000, 0.9129422336036122632 ) ) ;
#16794=VERTEX_POINT ( 'NONE', #9970 ) ;
#16803=EDGE_CURVE ( 'NONE', #7335, #15942, #15616, .T. ) ;
#16807=LINE ( 'NONE', #8718, #7243 ) ;
#16810=VERTEX_POINT ( 'NONE', #12411 ) ;
#16813=DIRECTION ( 'NONE',  ( 0.000000000000000000, -1.000000000000000000, -0.000000000000000000 ) ) ;
#16815=ADVANCED_FACE ( 'NONE', ( #17596 ), #7419, .T. ) ;
#16822=LINE ( 'NONE', #1342, #7746 ) ;
#16837=EDGE_CURVE ( 'NONE', #9905, #3908, #11425, .T. ) ;
#16840=LINE ( 'NONE', #11764, #6082 ) ;
#16843=ORIENTED_EDGE ( 'NONE', *, *, #7074, .F. ) ;
#16845=VECTOR ( 'NONE', #13172, 1000.000000000000114 ) ;
#16852=DIRECTION ( 'NONE',  ( 0.000000000000000000, 1.000000000000000000, 0.000000000000000000 ) ) ;
#16853=CARTESIAN_POINT ( 'NONE',  ( 42.79471501377724252, 34.52875999999999834, 5.049205022181460834 ) ) ;
#16855=ORIENTED_EDGE ( 'NONE', *, *, #17014, .F. ) ;
#16862=EDGE_CURVE ( 'NONE', #16009, #12286, #18446, .T. ) ;
#16864=ORIENTED_EDGE ( 'NONE', *, *, #19455, .T. ) ;
#16868=ORIENTED_EDGE ( 'NONE', *, *, #14301, .F. ) ;
#16873=DIRECTION ( 'NONE',  ( 0.000000000000000000, -1.000000000000000000, -0.000000000000000000 ) ) ;
#16874=ORIENTED_EDGE ( 'NONE', *, *, #12768, .F. ) ;
#16881=CARTESIAN_POINT ( 'NONE',  ( 37.13209340688868565, -6.356984999999999886, -3.529402718062123689 ) ) ;
#16885=ORIENTED_EDGE ( 'NONE', *, *, #9837, .T. ) ;
#16886=CARTESIAN_POINT ( 'NONE',  ( 56.91751438644678984, 34.52875999999999834, -20.96198986413465448 ) ) ;
#16889=DIRECTION ( 'NONE',  ( -0.6702301885068630005, 0.000000000000000000, -0.7421532822901580895 ) ) ;
#16899=ORIENTED_EDGE ( 'NONE', *, *, #5242, .F. ) ;
#16905=CARTESIAN_POINT ( 'NONE',  ( 60.38511073144201191, 32.54502000000000095, -22.26373525985038526 ) ) ;
#16909=B_SPLINE_CURVE_WITH_KNOTS ( 'NONE', 3,
 ( #19082, #4253, #930, #21475, #6452, #3246, #3362, #1254, #18180, #10090 ),
 .UNSPECIFIED., .F., .F.,
 ( 4, 2, 2, 2, 4 ),
 ( 0.003573252179933841116, 0.004059386830566638800, 0.004545521481199436484, 0.005031656131832235035, 0.005517790782465032719 ),
 .UNSPECIFIED. ) ;
#16913=CARTESIAN_POINT ( 'NONE',  ( 52.25311689352595579, -6.512906051756550241, -17.53621019291011152 ) ) ;
#16914=CARTESIAN_POINT ( 'NONE',  ( 32.42378190387104553, 0.000000000000000000, -18.15178106273469183 ) ) ;
#16917=CIRCLE ( 'NONE', #16156, 9.525000000000000355 ) ;
#16918=CARTESIAN_POINT ( 'NONE',  ( 52.44708915697334106, 34.52875999999999834, 4.020247972991190188 ) ) ;
#16924=AXIS2_PLACEMENT_3D ( 'NONE', #15184, #2452, #19249 ) ;
#16928=ADVANCED_FACE ( 'NONE', ( #12075 ), #2335, .T. ) ;
#16932=ADVANCED_FACE ( 'NONE', ( #19247 ), #10847, .T. ) ;
#16951=CARTESIAN_POINT ( 'NONE',  ( 49.13030338002142372, 109.3223030719999969, -2.154981381712871791 ) ) ;
#16953=LINE ( 'NONE', #16853, #2421 ) ;
#16954=CIRCLE ( 'NONE', #19427, 0.5080000000000005622 ) ;
#16958=EDGE_CURVE ( 'NONE', #5690, #11670, #18472, .T. ) ;
#16967=VECTOR ( 'NONE', #16873, 1000.000000000000000 ) ;
#16972=VERTEX_POINT ( 'NONE', #13152 ) ;
#16974=CARTESIAN_POINT ( 'NONE',  ( 47.80475250345343596, -5.166360000000002728, -11.91473563638196786 ) ) ;
#16977=VERTEX_POINT ( 'NONE', #19970 ) ;
#16982=ORIENTED_EDGE ( 'NONE', *, *, #4647, .T. ) ;
#16987=ORIENTED_EDGE ( 'NONE', *, *, #20989, .F. ) ;
#16988=CARTESIAN_POINT ( 'NONE',  ( 39.16413618835606769, 2.586003464000000029, -24.45043885672975392 ) ) ;
#16992=DIRECTION ( 'NONE',  ( -0.000000000000000000, -1.000000000000000000, 0.000000000000000000 ) ) ;
#16994=AXIS2_PLACEMENT_3D ( 'NONE', #10838, #17915, #17814 ) ;
#16996=CARTESIAN_POINT ( 'NONE',  ( 48.78323016782857735, 32.54502000000000095, -25.79158832643865651 ) ) ;
#17003=CIRCLE ( 'NONE', #4991, 0.5079999999999996740 ) ;
#17006=DIRECTION ( 'NONE',  ( -0.9943660382494290406, 0.000000000000000000, 0.1060008583745199739 ) ) ;
#17010=ORIENTED_EDGE ( 'NONE', *, *, #20701, .T. ) ;
#17014=EDGE_CURVE ( 'NONE', #6031, #17792, #7544, .T. ) ;
#17018=CARTESIAN_POINT ( 'NONE',  ( 34.84490081146155660, 0.000000000000000000, -0.2108409695808725060 ) ) ;
#17019=ADVANCED_FACE ( 'NONE', ( #18318, #21747 ), #9908, .T. ) ;
#17028=DIRECTION ( 'NONE',  ( 0.000000000000000000, 1.000000000000000000, 0.000000000000000000 ) ) ;
#17030=VERTEX_POINT ( 'NONE', #2560 ) ;
#17044=VECTOR ( 'NONE', #16076, 1000.000000000000000 ) ;
#17051=LINE ( 'NONE', #8415, #21547 ) ;
#17055=FACE_OUTER_BOUND ( 'NONE', #13031, .T. ) ;
#17058=CARTESIAN_POINT ( 'NONE',  ( 39.27728671717661513, 0.000000000000000000, -23.95520057284206672 ) ) ;
#17060=VERTEX_POINT ( 'NONE', #16674 ) ;
#17065=ORIENTED_EDGE ( 'NONE', *, *, #15233, .F. ) ;
#17068=CARTESIAN_POINT ( 'NONE',  ( 54.84114405289130900, -6.356984999999999886, -18.15059713109360473 ) ) ;
#17069=EDGE_CURVE ( 'NONE', #3974, #4463, #6877, .T. ) ;
#17072=EDGE_CURVE ( 'NONE', #1209, #14379, #9646, .T. ) ;
#17080=CARTESIAN_POINT ( 'NONE',  ( 52.79771328282338771, -1.983739999999999837, 3.317700572842066986 ) ) ;
#17082=LINE ( 'NONE', #6909, #10604 ) ;
#17095=AXIS2_PLACEMENT_3D ( 'NONE', #8768, #17185, #14932 ) ;
#17099=EDGE_CURVE ( 'NONE', #21489, #19201, #834, .T. ) ;
#17106=CARTESIAN_POINT ( 'NONE',  ( 42.66304184606194383, -9.531985000000000596, -19.22597499813143784 ) ) ;
#17121=EDGE_LOOP ( 'NONE', ( #981, #13175, #11729 ) ) ;
#17128=ORIENTED_EDGE ( 'NONE', *, *, #7000, .F. ) ;
#17133=EDGE_LOOP ( 'NONE', ( #7368, #3489, #15788, #5882 ) ) ;
#17138=DIRECTION ( 'NONE',  ( 0.000000000000000000, -1.000000000000000000, -0.000000000000000000 ) ) ;
#17142=CARTESIAN_POINT ( 'NONE',  ( 53.10651001381376091, -5.166360000000002728, -16.70269254552787075 ) ) ;
#17143=DIRECTION ( 'NONE',  ( 0.000000000000000000, -1.000000000000000000, -0.000000000000000000 ) ) ;
#17144=AXIS2_PLACEMENT_3D ( 'NONE', #20241, #5321, #3457 ) ;
#17148=DIRECTION ( 'NONE',  ( 0.000000000000000000, 1.000000000000000000, 0.000000000000000000 ) ) ;
#17168=EDGE_CURVE ( 'NONE', #8930, #6920, #8465, .T. ) ;
#17170=CARTESIAN_POINT ( 'NONE',  ( 61.02111788801703085, 34.52875999999999834, -5.406220493519755088 ) ) ;
#17175=VERTEX_POINT ( 'NONE', #18963 ) ;
#17185=DIRECTION ( 'NONE',  ( 0.000000000000000000, 1.000000000000000000, 0.000000000000000000 ) ) ;
#17190=EDGE_CURVE ( 'NONE', #7998, #2524, #5053, .T. ) ;
#17210=DIRECTION ( 'NONE',  ( 0.000000000000000000, 1.000000000000000000, -0.000000000000000000 ) ) ;
#17212=DIRECTION ( 'NONE',  ( 0.000000000000000000, 1.000000000000000000, 0.000000000000000000 ) ) ;
#17215=CARTESIAN_POINT ( 'NONE',  ( 43.29176983217143260, 34.52875999999999834, 5.154088326438659884 ) ) ;
#17219=LINE ( 'NONE', #8697, #21493 ) ;
#17222=ORIENTED_EDGE ( 'NONE', *, *, #4379, .T. ) ;
#17228=EDGE_CURVE ( 'NONE', #107, #1117, #2251, .T. ) ;
#17238=ADVANCED_FACE ( 'NONE', ( #2166 ), #12013, .F. ) ;
#17242=DIRECTION ( 'NONE',  ( -0.7532174416907910786, 0.000000000000000000, -0.6577716059034319773 ) ) ;
#17246=PRODUCT_DEFINITION_FORMATION_WITH_SPECIFIED_SOURCE ( 'ANY', '', #17286, .NOT_KNOWN. ) ;
#17248=DIRECTION ( 'NONE',  ( -0.3928209820863022839, 0.000000000000000000, 0.9196149607486564515 ) ) ;
#17249=CARTESIAN_POINT ( 'NONE',  ( 52.43369301778259484, -7.088958102700910757, -17.37753678331790397 ) ) ;
#17250=ORIENTED_EDGE ( 'NONE', *, *, #570, .T. ) ;
#17255=ORIENTED_EDGE ( 'NONE', *, *, #4953, .F. ) ;
#17277=FACE_OUTER_BOUND ( 'NONE', #8902, .T. ) ;
#17285=DIRECTION ( 'NONE',  ( 0.000000000000000000, -1.000000000000000000, -0.000000000000000000 ) ) ;
#17286=PRODUCT ( 'Split Webbing Winding Axle', 'Split Webbing Winding Axle', '', ( #12434 ) ) ;
#17296=CARTESIAN_POINT ( 'NONE',  ( 53.13667458378568398, -7.546788837613773282, -16.66913787414813086 ) ) ;
#17300=VERTEX_POINT ( 'NONE', #18634 ) ;
#17307=CIRCLE ( 'NONE', #13439, 30.16249999999999432 ) ;
#17310=ORIENTED_EDGE ( 'NONE', *, *, #1816, .F. ) ;
#17312=AXIS2_PLACEMENT_3D ( 'NONE', #4255, #12327, #15779 ) ;
#17315=CARTESIAN_POINT ( 'NONE',  ( 49.28028498622276032, -1.983739999999999837, -25.68670502218146368 ) ) ;
#17338=AXIS2_PLACEMENT_3D ( 'NONE', #11274, #2881, #9612 ) ;
#17351=EDGE_LOOP ( 'NONE', ( #21053, #3989, #9706, #15148 ) ) ;
#17352=ADVANCED_FACE ( 'NONE', ( #4175 ), #6261, .T. ) ;
#17354=AXIS2_PLACEMENT_3D ( 'NONE', #11465, #11567, #18305 ) ;
#17357=CARTESIAN_POINT ( 'NONE',  ( 38.27575909311416780, -6.969031819622845347, -4.797431545001941799 ) ) ;
#17372=ORIENTED_EDGE ( 'NONE', *, *, #21331, .F. ) ;
#17374=AXIS2_PLACEMENT_3D ( 'NONE', #2354, #690, #2010 ) ;
#17375=ORIENTED_EDGE ( 'NONE', *, *, #16277, .T. ) ;
#17377=TOROIDAL_SURFACE ( 'NONE', #4651, 3.174999999999999822, 1.190625000000000044 ) ;
#17386=CARTESIAN_POINT ( 'NONE',  ( 38.96848998618624904, 37.69740999999999786, -3.934807454472129429 ) ) ;
#17389=CIRCLE ( 'NONE', #18083, 1.190625000000000711 ) ;
#17393=CIRCLE ( 'NONE', #781, 0.5080000000000016724 ) ;
#17397=CARTESIAN_POINT ( 'NONE',  ( 64.19677489640052670, 29.95901653600000003, -11.74367670905533423 ) ) ;
#17400=VECTOR ( 'NONE', #12893, 1000.000000000000000 ) ;
#17404=CARTESIAN_POINT ( 'NONE',  ( 57.69402548289047417, 0.000000000000000000, -20.84562559047711261 ) ) ;
#17408=VERTEX_POINT ( 'NONE', #6043 ) ;
#17410=AXIS2_PLACEMENT_3D ( 'NONE', #16421, #9981, #8318 ) ;
#17412=VECTOR ( 'NONE', #20097, 1000.000000000000000 ) ;
#17413=ORIENTED_EDGE ( 'NONE', *, *, #11325, .F. ) ;
#17418=DIRECTION ( 'NONE',  ( 0.000000000000000000, -1.000000000000000000, -0.000000000000000000 ) ) ;
#17424=CYLINDRICAL_SURFACE ( 'NONE', #10926, 0.5080000000000001181 ) ;
#17429=CIRCLE ( 'NONE', #12851, 0.5080000000000012284 ) ;
#17432=CARTESIAN_POINT ( 'NONE',  ( 49.72033008250774344, -1.983739999999999837, -2.687827786179598277 ) ) ;
#17446=CYLINDRICAL_SURFACE ( 'NONE', #1867, 0.5079999999999984528 ) ;
#17449=AXIS2_PLACEMENT_3D ( 'NONE', #8854, #19020, #7097 ) ;
#17452=ADVANCED_FACE ( 'NONE', ( #21298 ), #12925, .F. ) ;
#17474=DIRECTION ( 'NONE',  ( 0.000000000000000000, 1.000000000000000000, 0.000000000000000000 ) ) ;
#17480=LINE ( 'NONE', #13649, #20337 ) ;
#17488=LINE ( 'NONE', #2331, #9071 ) ;
#17494=EDGE_CURVE ( 'NONE', #4294, #9387, #6018, .T. ) ;
#17501=DIRECTION ( 'NONE',  ( -0.3542738219355860418, 0.000000000000000000, -0.9351417320872557060 ) ) ;
#17504=CYLINDRICAL_SURFACE ( 'NONE', #15244, 0.5080000000000000071 ) ;
#17512=CARTESIAN_POINT ( 'NONE',  ( 37.09580597189848561, 38.88803500000000213, 2.672127428255844261 ) ) ;
#17518=VERTEX_POINT ( 'NONE', #10020 ) ;
#17526=CARTESIAN_POINT ( 'NONE',  ( 48.78323016782857735, 34.52875999999999834, -25.79158832643865651 ) ) ;
#17529=ORIENTED_EDGE ( 'NONE', *, *, #14301, .T. ) ;
#17536=DIRECTION ( 'NONE',  ( -0.3542738219355860418, 0.000000000000000000, -0.9351417320872557060 ) ) ;
#17542=CARTESIAN_POINT ( 'NONE',  ( 38.96848998618624904, -7.547609999999999708, -3.934807454472129429 ) ) ;
#17547=EDGE_LOOP ( 'NONE', ( #485, #11061, #20777, #1287 ) ) ;
#17548=CARTESIAN_POINT ( 'NONE',  ( 32.55306802826559220, 34.52875999999999834, -17.37731658638881527 ) ) ;
#17550=DIRECTION ( 'NONE',  ( -0.000000000000000000, -1.000000000000000000, 0.000000000000000000 ) ) ;
#17555=ORIENTED_EDGE ( 'NONE', *, *, #5447, .F. ) ;
#17559=VERTEX_POINT ( 'NONE', #58 ) ;
#17565=VERTEX_POINT ( 'NONE', #20060 ) ;
#17566=AXIS2_PLACEMENT_3D ( 'NONE', #3509, #7272, #3736 ) ;
#17568=ORIENTED_EDGE ( 'NONE', *, *, #15268, .F. ) ;
#17575=ORIENTED_EDGE ( 'NONE', *, *, #21140, .T. ) ;
#17581=VERTEX_POINT ( 'NONE', #19963 ) ;
#17585=DIRECTION ( 'NONE',  ( -0.4987171968201988270, 0.000000000000000000, 0.8667647648559574369 ) ) ;
#17589=ORIENTED_EDGE ( 'NONE', *, *, #12995, .T. ) ;
#17590=CARTESIAN_POINT ( 'NONE',  ( 44.27024749654656688, -9.531985000000000596, -8.722764363618033201 ) ) ;
#17593=DIRECTION ( 'NONE',  ( 0.1060008583745224581, 0.000000000000000000, 0.9943660382494288186 ) ) ;
#17596=FACE_OUTER_BOUND ( 'NONE', #1970, .T. ) ;
#17597=EDGE_CURVE ( 'NONE', #723, #18266, #3165, .T. ) ;
#17613=CARTESIAN_POINT ( 'NONE',  ( 49.41195815393805901, 42.06303499999999929, -1.411525001868561224 ) ) ;
#17622=EDGE_CURVE ( 'NONE', #21599, #7945, #15570, .T. ) ;
#17623=VECTOR ( 'NONE', #9358, 1000.000000000000114 ) ;
#17626=EDGE_CURVE ( 'NONE', #5142, #13568, #2640, .T. ) ;
#17629=FACE_OUTER_BOUND ( 'NONE', #20350, .T. ) ;
#17632=CARTESIAN_POINT ( 'NONE',  ( 53.10651001381376091, -5.166360000000002728, -16.70269254552787075 ) ) ;
#17633=ORIENTED_EDGE ( 'NONE', *, *, #12053, .F. ) ;
#17635=DIRECTION ( 'NONE',  ( 0.000000000000000000, 1.000000000000000000, 0.000000000000000000 ) ) ;
#17636=VERTEX_POINT ( 'NONE', #20721 ) ;
#17644=DIRECTION ( 'NONE',  ( 1.000000000000000000, 0.000000000000000000, 0.000000000000000000 ) ) ;
#17645=ADVANCED_FACE ( 'NONE', ( #15559 ), #2153, .F. ) ;
#17659=DIRECTION ( 'NONE',  ( 0.000000000000000000, -1.000000000000000000, -0.000000000000000000 ) ) ;
#17661=DIRECTION ( 'NONE',  ( 0.000000000000000000, 1.000000000000000000, 0.000000000000000000 ) ) ;
#17666=ORIENTED_EDGE ( 'NONE', *, *, #12659, .T. ) ;
#17667=CARTESIAN_POINT ( 'NONE',  ( 46.03750000000000142, 42.06303499999999929, -10.31874999999999964 ) ) ;
#17678=VECTOR ( 'NONE', #7428, 1000.000000000000000 ) ;
#17688=LINE ( 'NONE', #2539, #15275 ) ;
#17693=VERTEX_POINT ( 'NONE', #611 ) ;
#17699=VERTEX_POINT ( 'NONE', #14124 ) ;
#17707=CIRCLE ( 'NONE', #17354, 1.190624999999997824 ) ;
#17710=LINE ( 'NONE', #7218, #2104 ) ;
#17718=DIRECTION ( 'NONE',  ( 0.000000000000000000, 1.000000000000000000, 0.000000000000000000 ) ) ;
#17721=CIRCLE ( 'NONE', #17374, 0.7950199999999985057 ) ;
#17722=ORIENTED_EDGE ( 'NONE', *, *, #13591, .F. ) ;
#17723=DIRECTION ( 'NONE',  ( 0.05085730733808139364, 0.000000000000000000, -0.9987059298363658577 ) ) ;
#17725=VECTOR ( 'NONE', #20775, 1000.000000000000114 ) ;
#17727=ORIENTED_EDGE ( 'NONE', *, *, #21824, .T. ) ;
#17737=CARTESIAN_POINT ( 'NONE',  ( 42.94469661997857912, 34.52875999999999834, -18.48251861828712705 ) ) ;
#17746=CARTESIAN_POINT ( 'NONE',  ( 39.58386072796507449, 37.69740999999999786, -4.490541772578644064 ) ) ;
#17747=DIRECTION ( 'NONE',  ( 0.000000000000000000, 1.000000000000000000, 0.000000000000000000 ) ) ;
#17750=DIRECTION ( 'NONE',  ( 0.000000000000000000, 1.000000000000000000, 0.000000000000000000 ) ) ;
#17766=CARTESIAN_POINT ( 'NONE',  ( 39.64083910660897203, -7.089776582593554366, -3.260385504968207115 ) ) ;
#17771=EDGE_LOOP ( 'NONE', ( #19707, #11950, #4371, #15425 ) ) ;
#17772=CARTESIAN_POINT ( 'NONE',  ( 47.80475250345343596, 38.88803500000000213, -11.91473563638196786 ) ) ;
#17778=VERTEX_POINT ( 'NONE', #20491 ) ;
#17779=CARTESIAN_POINT ( 'NONE',  ( 42.79471501377724252, -1.983739999999999837, 5.049205022181460834 ) ) ;
#17780=CARTESIAN_POINT ( 'NONE',  ( 38.28489021960990613, 38.88803500000000213, 2.732679409805250703 ) ) ;
#17789=ORIENTED_EDGE ( 'NONE', *, *, #1271, .T. ) ;
#17792=VERTEX_POINT ( 'NONE', #13911 ) ;
#17793=ORIENTED_EDGE ( 'NONE', *, *, #11625, .T. ) ;
#17800=DIRECTION ( 'NONE',  ( 0.000000000000000000, 1.000000000000000000, 0.000000000000000000 ) ) ;
#17805=CARTESIAN_POINT ( 'NONE',  ( 49.15122309515935228, 34.52875999999999834, -25.07506492104907991 ) ) ;
#17806=DIRECTION ( 'NONE',  ( -0.1060008583745224581, 0.000000000000000000, -0.9943660382494288186 ) ) ;
#17810=ORIENTED_EDGE ( 'NONE', *, *, #16577, .T. ) ;
#17813=DIRECTION ( 'NONE',  ( -0.4080888115384288528, 0.000000000000000000, -0.9129422336036122632 ) ) ;
#17814=DIRECTION ( 'NONE',  ( 0.05085730733808142834, 0.000000000000000000, -0.9987059298363657467 ) ) ;
#17815=AXIS2_PLACEMENT_3D ( 'NONE', #8942, #9265, #19109 ) ;
#17817=ORIENTED_EDGE ( 'NONE', *, *, #7822, .F. ) ;
#17822=CARTESIAN_POINT ( 'NONE',  ( 59.55063415577301811, 32.54502000000000095, -22.52230776719629191 ) ) ;
#17824=VECTOR ( 'NONE', #16422, 1000.000000000000114 ) ;
#17836=CARTESIAN_POINT ( 'NONE',  ( 53.09010322336158794, 40.07841907356969813, -16.72081503543966718 ) ) ;
#17841=CARTESIAN_POINT ( 'NONE',  ( 44.27024749654656688, 38.88803500000000213, -8.722764363618033201 ) ) ;
#17856=DIRECTION ( 'NONE',  ( -0.4987171968201928873, 0.000000000000000000, 0.8667647648559606566 ) ) ;
#17858=DIRECTION ( 'NONE',  ( 0.000000000000000000, 1.000000000000000000, 0.000000000000000000 ) ) ;
#17872=CARTESIAN_POINT ( 'NONE',  ( 39.07402576619974610, -5.166360000000001840, -3.817946520901574825 ) ) ;
#17880=EDGE_CURVE ( 'NONE', #16009, #18389, #2938, .T. ) ;
#17881=CARTESIAN_POINT ( 'NONE',  ( 38.95212789349618987, -7.547369073570063591, -3.952970310398209897 ) ) ;
#17884=DIRECTION ( 'NONE',  ( -0.9987059298363656357, 0.000000000000000000, -0.05085730733808393328 ) ) ;
#17886=ORIENTED_EDGE ( 'NONE', *, *, #1430, .T. ) ;
#17892=EDGE_LOOP ( 'NONE', ( #12128, #14615, #15949, #14945 ) ) ;
#17894=EDGE_CURVE ( 'NONE', #1735, #19311, #9988, .T. ) ;
#17898=CARTESIAN_POINT ( 'NONE',  ( 30.25543876212147509, 0.000000000000000000, -19.39939755251907272 ) ) ;
#17904=FACE_OUTER_BOUND ( 'NONE', #14637, .T. ) ;
#17906=FACE_OUTER_BOUND ( 'NONE', #16103, .T. ) ;
#17909=B_SPLINE_CURVE_WITH_KNOTS ( 'NONE', 3,
 ( #5718, #2403, #6151, #17881, #19200 ),
 .UNSPECIFIED., .F., .F.,
 ( 4, 1, 4 ),
 ( 0.003754349818373690570, 0.003769101685636799468, 0.003783853552899908799 ),
 .UNSPECIFIED. ) ;
#17911=ORIENTED_EDGE ( 'NONE', *, *, #1634, .F. ) ;
#17913=AXIS2_PLACEMENT_3D ( 'NONE', #20203, #9716, #1636 ) ;
#17915=DIRECTION ( 'NONE',  ( -0.9987059298363656357, 0.000000000000000000, -0.05085730733808393328 ) ) ;
#17917=ORIENTED_EDGE ( 'NONE', *, *, #9837, .F. ) ;
#17918=ORIENTED_EDGE ( 'NONE', *, *, #3436, .F. ) ;
#17919=DIRECTION ( 'NONE',  ( 0.7421532822901580895, -0.000000000000000000, -0.6702301885068630005 ) ) ;
#17930=CARTESIAN_POINT ( 'NONE',  ( 42.35466991749225940, 34.52876000000000545, -17.94967221382040279 ) ) ;
#17936=CARTESIAN_POINT ( 'NONE',  ( 39.16413618835606769, -1.983739999999999837, -24.45043885672975392 ) ) ;
#17939=CARTESIAN_POINT ( 'NONE',  ( 53.25483508941461963, -9.531985000000000596, -5.879799058943532941 ) ) ;
#17953=DIRECTION ( 'NONE',  ( -0.6702301885068639997, 0.000000000000000000, -0.7421532822901570903 ) ) ;
#17957=AXIS2_PLACEMENT_3D ( 'NONE', #895, #9066, #18909 ) ;
#17959=CARTESIAN_POINT ( 'NONE',  ( 59.90456643211351917, 34.52875999999999834, -2.926035437812116946 ) ) ;
#17966=ORIENTED_EDGE ( 'NONE', *, *, #597, .T. ) ;
#17971=DIRECTION ( 'NONE',  ( 0.000000000000000000, 1.000000000000000000, -0.000000000000000000 ) ) ;
#17974=EDGE_CURVE ( 'NONE', #1074, #13360, #8225, .T. ) ;
#17986=ORIENTED_EDGE ( 'NONE', *, *, #4111, .F. ) ;
#17990=DIRECTION ( 'NONE',  ( 0.000000000000000000, -1.000000000000000000, -0.000000000000000000 ) ) ;
#17993=CIRCLE ( 'NONE', #16924, 1.190625000000001155 ) ;
#17996=ORIENTED_EDGE ( 'NONE', *, *, #2193, .T. ) ;
#18005=EDGE_LOOP ( 'NONE', ( #4696, #400 ) ) ;
#18011=DIRECTION ( 'NONE',  ( 0.9129422336036140395, 0.000000000000000000, -0.4080888115384250225 ) ) ;
#18012=ORIENTED_EDGE ( 'NONE', *, *, #10925, .T. ) ;
#18016=CARTESIAN_POINT ( 'NONE',  ( 39.62791084302666178, 32.54502000000000095, -24.65774797299118859 ) ) ;
#18017=DIRECTION ( 'NONE',  ( -0.7421532822901580895, 0.000000000000000000, 0.6702301885068630005 ) ) ;
#18019=VERTEX_POINT ( 'NONE', #19937 ) ;
#18023=ADVANCED_FACE ( 'NONE', ( #3662, #11542 ), #10407, .T. ) ;
#18031=DIRECTION ( 'NONE',  ( 0.000000000000000000, -1.000000000000000000, -0.000000000000000000 ) ) ;
#18034=DIRECTION ( 'NONE',  ( 0.000000000000000000, -1.000000000000000000, -0.000000000000000000 ) ) ;
#18035=VERTEX_POINT ( 'NONE', #11650 ) ;
#18038=DIRECTION ( 'NONE',  ( 0.000000000000000000, 1.000000000000000000, 0.000000000000000000 ) ) ;
#18042=VERTEX_POINT ( 'NONE', #6569 ) ;
#18047=AXIS2_PLACEMENT_3D ( 'NONE', #21722, #15004, #34 ) ;
#18049=AXIS2_PLACEMENT_3D ( 'NONE', #16221, #21387, #16111 ) ;
#18051=FACE_OUTER_BOUND ( 'NONE', #21296, .T. ) ;
#18063=CARTESIAN_POINT ( 'NONE',  ( 31.68988926855799448, -1.983739999999999837, 1.626235259850384418 ) ) ;
#18065=CARTESIAN_POINT ( 'NONE',  ( 39.11079947626275555, 34.52875999999999834, -27.65534212225540500 ) ) ;
#18072=AXIS2_PLACEMENT_3D ( 'NONE', #11840, #3540, #21677 ) ;
#18076=VERTEX_POINT ( 'NONE', #3041 ) ;
#18080=FACE_OUTER_BOUND ( 'NONE', #21596, .T. ) ;
#18081=ORIENTED_EDGE ( 'NONE', *, *, #12249, .T. ) ;
#18083=AXIS2_PLACEMENT_3D ( 'NONE', #3758, #14374, #20993 ) ;
#18091=CIRCLE ( 'NONE', #4676, 0.7950199999999982836 ) ;
#18093=CARTESIAN_POINT ( 'NONE',  ( 38.36471077000297925, 38.15731773671534910, -4.673719963191772742 ) ) ;
#18101=CARTESIAN_POINT ( 'NONE',  ( 53.14266576735298031, -7.546379553159687781, -16.66242751532464084 ) ) ;
#18103=ORIENTED_EDGE ( 'NONE', *, *, #6811, .T. ) ;
#18106=AXIS2_PLACEMENT_3D ( 'NONE', #625, #4164, #7369 ) ;
#18108=CARTESIAN_POINT ( 'NONE',  ( 60.38511073144201191, 32.54502000000000095, -22.26373525985038526 ) ) ;
#18114=AXIS2_PLACEMENT_3D ( 'NONE', #11592, #80, #1627 ) ;
#18117=AXIS2_PLACEMENT_3D ( 'NONE', #18485, #5112, #11860 ) ;
#18119=LINE ( 'NONE', #874, #6156 ) ;
#18123=EDGE_CURVE ( 'NONE', #14487, #14185, #19399, .T. ) ;
#18128=CARTESIAN_POINT ( 'NONE',  ( 53.31277592387545639, 40.04741288645178088, -16.46826747127406421 ) ) ;
#18129=AXIS2_PLACEMENT_3D ( 'NONE', #17215, #2058, #5599 ) ;
#18131=ORIENTED_EDGE ( 'NONE', *, *, #17626, .T. ) ;
#18133=CARTESIAN_POINT ( 'NONE',  ( 54.55586098912687731, -9.531985000000000596, -6.056925149195119040 ) ) ;
#18135=EDGE_LOOP ( 'NONE', ( #12369, #8060, #530, #17789 ) ) ;
#18138=B_SPLINE_CURVE_WITH_KNOTS ( 'NONE', 3,
 ( #3814, #3184, #11481, #17296, #499 ),
 .UNSPECIFIED., .F., .F.,
 ( 4, 1, 4 ),
 ( 0.000000000000000000, 2.695145556491273853E-05, 5.390291112982547705E-05 ),
 .UNSPECIFIED. ) ;
#18149=EDGE_CURVE ( 'NONE', #8377, #7695, #5646, .T. ) ;
#18152=VERTEX_POINT ( 'NONE', #17930 ) ;
#18172=EDGE_CURVE ( 'NONE', #10096, #3095, #14480, .T. ) ;
#18176=CARTESIAN_POINT ( 'NONE',  ( 61.65536943582333151, 32.54502000000000095, -11.98363747855214712 ) ) ;
#18178=CARTESIAN_POINT ( 'NONE',  ( 51.69314645384351081, -6.356984999999999886, -17.03058447914853346 ) ) ;
#18180=CARTESIAN_POINT ( 'NONE',  ( 39.11418302930122337, 40.08456717457784890, -3.775083184656583768 ) ) ;
#18182=LINE ( 'NONE', #3134, #13802 ) ;
#18185=DIRECTION ( 'NONE',  ( -0.7421532822901579785, 0.000000000000000000, 0.6702301885068630005 ) ) ;
#18186=ORIENTED_EDGE ( 'NONE', *, *, #620, .T. ) ;
#18189=CARTESIAN_POINT ( 'NONE',  ( 52.19854938732527216, 38.72945808962413849, -17.58284632693144189 ) ) ;
#18191=CARTESIAN_POINT ( 'NONE',  ( 50.29383871662588490, -4.569743463999999200, -28.02957329025317179 ) ) ;
#18196=ORIENTED_EDGE ( 'NONE', *, *, #8436, .F. ) ;
#18198=EDGE_CURVE ( 'NONE', #5911, #2030, #19046, .T. ) ;
#18202=EDGE_LOOP ( 'NONE', ( #21287, #16557, #4055, #12617 ) ) ;
#18204=CARTESIAN_POINT ( 'NONE',  ( 38.31336037684268092, 38.28835795706343958, -4.744980486405671272 ) ) ;
#18209=ORIENTED_EDGE ( 'NONE', *, *, #15387, .T. ) ;
#18221=DIRECTION ( 'NONE',  ( -0.7532174416907910786, 0.000000000000000000, -0.6577716059034319773 ) ) ;
#18225=LINE ( 'NONE', #3082, #4402 ) ;
#18228=ORIENTED_EDGE ( 'NONE', *, *, #17072, .F. ) ;
#18230=CARTESIAN_POINT ( 'NONE',  ( 43.47225467835599488, 38.88803500000000213, -9.606390615344288619 ) ) ;
#18237=EDGE_LOOP ( 'NONE', ( #7498, #10131, #17575, #3069 ) ) ;
#18239=DIRECTION ( 'NONE',  ( 0.000000000000000000, -1.000000000000000000, -0.000000000000000000 ) ) ;
#18245=AXIS2_PLACEMENT_3D ( 'NONE', #4098, #2437, #17585 ) ;
#18246=ORIENTED_EDGE ( 'NONE', *, *, #15074, .T. ) ;
#18263=AXIS2_PLACEMENT_3D ( 'NONE', #10742, #784, #15840 ) ;
#18265=CARTESIAN_POINT ( 'NONE',  ( 38.82016491058538321, 32.54502000000000095, -14.75770094105646812 ) ) ;
#18266=VERTEX_POINT ( 'NONE', #1223 ) ;
#18268=CARTESIAN_POINT ( 'NONE',  ( 38.32982792479189271, -5.610959413415746333, -4.721377477347955320 ) ) ;
#18273=CARTESIAN_POINT ( 'NONE',  ( 59.90456643211351917, 0.000000000000000000, -2.926035437812116946 ) ) ;
#18278=ADVANCED_FACE ( 'NONE', ( #12742 ), #6300, .T. ) ;
#18279=CARTESIAN_POINT ( 'NONE',  ( 54.55586098912687731, 0.000000000000000000, -6.056925149195119040 ) ) ;
#18290=EDGE_CURVE ( 'NONE', #3524, #18035, #5868, .T. ) ;
#18304=ADVANCED_FACE ( 'NONE', ( #7750 ), #21232, .T. ) ;
#18305=DIRECTION ( 'NONE',  ( -0.9987059298363657467, 0.000000000000000000, -0.05085730733808409287 ) ) ;
#18308=ADVANCED_FACE ( 'NONE', ( #13801 ), #8067, .F. ) ;
#18318=FACE_OUTER_BOUND ( 'NONE', #6748, .T. ) ;
#18324=DIRECTION ( 'NONE',  ( -0.6702301885068628895, 0.000000000000000000, -0.7421532822901579785 ) ) ;
#18326=ORIENTED_EDGE ( 'NONE', *, *, #19101, .T. ) ;
#18330=ADVANCED_FACE ( 'NONE', ( #15247 ), #21558, .T. ) ;
#18333=EDGE_CURVE ( 'NONE', #10995, #20322, #185, .T. ) ;
#18336=LINE ( 'NONE', #6402, #16845 ) ;
#18340=ORIENTED_EDGE ( 'NONE', *, *, #21504, .T. ) ;
#18343=CARTESIAN_POINT ( 'NONE',  ( 53.69636427252483202, 38.88803500000000213, -18.48840734645144224 ) ) ;
#18346=CARTESIAN_POINT ( 'NONE',  ( 53.00421038040393995, -1.983739999999999837, 6.511420152579801446 ) ) ;
#18347=AXIS2_PLACEMENT_3D ( 'NONE', #9557, #16434, #13118 ) ;
#18349=APPLICATION_CONTEXT ( 'automotive_design' ) ;
#18355=EDGE_CURVE ( 'NONE', #19859, #4163, #13692, .T. ) ;
#18360=COLOUR_RGB ( '', 0.08235294, 0.09019608, 0.10196078) ;
#18362=DIRECTION ( 'NONE',  ( 0.000000000000000000, -1.000000000000000000, -0.000000000000000000 ) ) ;
#18366=DIRECTION ( 'NONE',  ( 0.000000000000000000, -1.000000000000000000, -0.000000000000000000 ) ) ;
#18367=DIRECTION ( 'NONE',  ( 0.000000000000000000, 1.000000000000000000, 0.000000000000000000 ) ) ;
#18373=DIRECTION ( 'NONE',  ( 0.000000000000000000, -1.000000000000000000, -0.000000000000000000 ) ) ;
#18382=CARTESIAN_POINT ( 'NONE',  ( 59.65121809612895731, 0.000000000000000000, -2.485718937265306572 ) ) ;
#18389=VERTEX_POINT ( 'NONE', #8471 ) ;
#18394=AXIS2_PLACEMENT_3D ( 'NONE', #16951, #20039, #13547 ) ;
#18395=AXIS2_PLACEMENT_3D ( 'NONE', #6258, #9787, #21509 ) ;
#18399=ADVANCED_FACE ( 'NONE', ( #15469 ), #3505, .T. ) ;
#18400=CARTESIAN_POINT ( 'NONE',  ( 38.49896492022744354, 37.93513121111498521, -4.495645369696349647 ) ) ;
#18406=EDGE_CURVE ( 'NONE', #8918, #8259, #11294, .T. ) ;
#18416=AXIS2_PLACEMENT_3D ( 'NONE', #19901, #12973, #7863 ) ;
#18417=AXIS2_PLACEMENT_3D ( 'NONE', #1099, #9607, #10941 ) ;
#18421=EDGE_LOOP ( 'NONE', ( #4568, #4638, #14477 ) ) ;
#18427=DIRECTION ( 'NONE',  ( 0.000000000000000000, 1.000000000000000000, 0.000000000000000000 ) ) ;
#18428=VERTEX_POINT ( 'NONE', #8688 ) ;
#18430=TOROIDAL_SURFACE ( 'NONE', #11735, 3.174999999999999822, 1.190625000000000044 ) ;
#18432=CIRCLE ( 'NONE', #14583, 30.16249999999998366 ) ;
#18433=LINE ( 'NONE', #1623, #18786 ) ;
#18437=AXIS2_PLACEMENT_3D ( 'NONE', #5712, #9349, #7482 ) ;
#18440=DIRECTION ( 'NONE',  ( 0.000000000000000000, 1.000000000000000000, 0.000000000000000000 ) ) ;
#18441=FACE_OUTER_BOUND ( 'NONE', #21872, .T. ) ;
#18443=VERTEX_POINT ( 'NONE', #6715 ) ;
#18446=B_SPLINE_CURVE_WITH_KNOTS ( 'NONE', 3,
 ( #18912, #20561, #10517, #15960, #12189 ),
 .UNSPECIFIED., .F., .F.,
 ( 4, 1, 4 ),
 ( 0.000000000000000000, 2.695145555969153257E-05, 5.390291111938306514E-05 ),
 .UNSPECIFIED. ) ;
#18456=EDGE_CURVE ( 'NONE', #11378, #13886, #20392, .T. ) ;
#18457=EDGE_CURVE ( 'NONE', #15003, #2583, #14854, .T. ) ;
#18460=AXIS2_PLACEMENT_3D ( 'NONE', #15041, #18642, #5162 ) ;
#18461=CARTESIAN_POINT ( 'NONE',  ( 41.78116128337411794, 32.54502000000000095, 7.392073290253172502 ) ) ;
#18466=FACE_OUTER_BOUND ( 'NONE', #747, .T. ) ;
#18467=CARTESIAN_POINT ( 'NONE',  ( 52.59520707473905787, -7.308466495983068967, -17.22774659103923156 ) ) ;
#18470=VERTEX_POINT ( 'NONE', #15572 ) ;
#18472=CIRCLE ( 'NONE', #19227, 0.5080000000000002292 ) ;
#18474=ORIENTED_EDGE ( 'NONE', *, *, #10660, .T. ) ;
#18477=DIRECTION ( 'NONE',  ( 0.8583349619704310207, 0.000000000000000000, -0.5130897514657826175 ) ) ;
#18482=AXIS2_PLACEMENT_3D ( 'NONE', #20387, #1941, #1725 ) ;
#18485=CARTESIAN_POINT ( 'NONE',  ( 27.87822510359947614, 32.54502000000000095, -8.893823290944665061 ) ) ;
#18486=LINE ( 'NONE', #2927, #9610 ) ;
#18488=DIRECTION ( 'NONE',  ( 0.9943660382494290406, 0.000000000000000000, -0.1060008583745199739 ) ) ;
#18492=ORIENTED_EDGE ( 'NONE', *, *, #8938, .F. ) ;
#18498=DIRECTION ( 'NONE',  ( 0.000000000000000000, -1.000000000000000000, -0.000000000000000000 ) ) ;
#18504=DIRECTION ( 'NONE',  ( -0.6702301885068639997, 0.000000000000000000, -0.7421532822901570903 ) ) ;
#18506=AXIS2_PLACEMENT_3D ( 'NONE', #13668, #20370, #5234 ) ;
#18507=EDGE_CURVE ( 'NONE', #1126, #19175, #10424, .T. ) ;
#18509=ORIENTED_EDGE ( 'NONE', *, *, #2816, .F. ) ;
#18518=CARTESIAN_POINT ( 'NONE',  ( 53.00421038040393995, 34.52875999999999834, 6.511420152579801446 ) ) ;
#18519=ORIENTED_EDGE ( 'NONE', *, *, #14653, .F. ) ;
#18523=CIRCLE ( 'NONE', #20991, 30.16249999999999787 ) ;
#18526=CARTESIAN_POINT ( 'NONE',  ( 53.13666646117270886, -5.167180607494337607, -16.66914697179084826 ) ) ;
#18533=EDGE_CURVE ( 'NONE', #16034, #19608, #2117, .T. ) ;
#18535=ORIENTED_EDGE ( 'NONE', *, *, #3143, .T. ) ;
#18536=ADVANCED_FACE ( 'NONE', ( #5212 ), #5003, .T. ) ;
#18537=CIRCLE ( 'NONE', #9006, 0.5079999999999984528 ) ;
#18541=DIRECTION ( 'NONE',  ( 0.000000000000000000, 1.000000000000000000, 0.000000000000000000 ) ) ;
#18544=CARTESIAN_POINT ( 'NONE',  ( 36.73521423675246922, 32.54502000000000095, 2.413462327205186497 ) ) ;
#18546=LINE ( 'NONE', #5384, #7143 ) ;
#18551=ORIENTED_EDGE ( 'NONE', *, *, #18805, .T. ) ;
#18555=EDGE_CURVE ( 'NONE', #18960, #17030, #17051, .T. ) ;
#18564=DIRECTION ( 'NONE',  ( -0.7421532822901579785, 0.000000000000000000, 0.6702301885068628895 ) ) ;
#18566=DIRECTION ( 'NONE',  ( 0.9129422336036140395, 0.000000000000000000, -0.4080888115384250225 ) ) ;
#18570=CARTESIAN_POINT ( 'NONE',  ( 59.89111109153450485, -4.569743463999999200, -22.14529389979288965 ) ) ;
#18571=CARTESIAN_POINT ( 'NONE',  ( 53.25483508941461963, -9.531985000000000596, -5.879799058943532941 ) ) ;
#18572=DIRECTION ( 'NONE',  ( 0.000000000000000000, 1.000000000000000000, 0.000000000000000000 ) ) ;
#18573=ORIENTED_EDGE ( 'NONE', *, *, #10758, .T. ) ;
#18579=EDGE_CURVE ( 'NONE', #119, #13886, #7426, .T. ) ;
#18593=EDGE_LOOP ( 'NONE', ( #9732, #753, #9492, #17886 ) ) ;
#18596=CARTESIAN_POINT ( 'NONE',  ( 38.28489021960990613, 38.88803500000000213, 2.732679409805250703 ) ) ;
#18598=VERTEX_POINT ( 'NONE', #3902 ) ;
#18601=AXIS2_PLACEMENT_3D ( 'NONE', #15799, #12919, #4396 ) ;
#18605=ORIENTED_EDGE ( 'NONE', *, *, #18507, .T. ) ;
#18617=DIRECTION ( 'NONE',  ( 0.000000000000000000, 1.000000000000000000, 0.000000000000000000 ) ) ;
#18619=ORIENTED_EDGE ( 'NONE', *, *, #10660, .F. ) ;
#18624=EDGE_CURVE ( 'NONE', #10134, #13027, #13099, .T. ) ;
#18625=CARTESIAN_POINT ( 'NONE',  ( 49.13030338002142372, -1.983739999999999837, -2.154981381712871791 ) ) ;
#18629=ORIENTED_EDGE ( 'NONE', *, *, #13340, .F. ) ;
#18634=CARTESIAN_POINT ( 'NONE',  ( 27.40895291499714403, -1.983739999999999837, -9.088367920799473865 ) ) ;
#18636=DIRECTION ( 'NONE',  ( 0.000000000000000000, -1.000000000000000000, -0.000000000000000000 ) ) ;
#18637=CARTESIAN_POINT ( 'NONE',  ( 30.97944403357121956, 34.52875999999999834, -8.103300075789407586 ) ) ;
#18638=DIRECTION ( 'NONE',  ( 0.9237641507921645623, 0.000000000000000000, 0.3829618697876213673 ) ) ;
#18642=DIRECTION ( 'NONE',  ( 0.000000000000000000, 1.000000000000000000, -0.000000000000000000 ) ) ;
#18645=CARTESIAN_POINT ( 'NONE',  ( 27.40895291499714403, 0.000000000000000000, -9.088367920799473865 ) ) ;
#18646=DIRECTION ( 'NONE',  ( 0.000000000000000000, 1.000000000000000000, 0.000000000000000000 ) ) ;
#18648=ORIENTED_EDGE ( 'NONE', *, *, #13057, .F. ) ;
#18652=AXIS2_PLACEMENT_3D ( 'NONE', #12287, #5303, #1992 ) ;
#18663=FACE_OUTER_BOUND ( 'NONE', #17121, .T. ) ;
#18666=CARTESIAN_POINT ( 'NONE',  ( 30.24348838687780727, 32.54502000000000095, -20.27293523655082552 ) ) ;
#18669=CARTESIAN_POINT ( 'NONE',  ( 61.09555596642878328, 32.54502000000000095, -12.53419992421059348 ) ) ;
#18670=CARTESIAN_POINT ( 'NONE',  ( 52.43275354619881057, -5.626267736715355738, -17.37840939435159981 ) ) ;
#18672=EDGE_CURVE ( 'NONE', #19005, #6777, #3, .T. ) ;
#18674=AXIS2_PLACEMENT_3D ( 'NONE', #12563, #17635, #21157 ) ;
#18675=EDGE_CURVE ( 'NONE', #6476, #12607, #3790, .T. ) ;
#18678=EDGE_LOOP ( 'NONE', ( #12002, #1973, #21539 ) ) ;
#18691=EDGE_CURVE ( 'NONE', #9393, #8373, #8128, .T. ) ;
#18694=CARTESIAN_POINT ( 'NONE',  ( 47.80475250345301674, -6.356984999999999886, -11.91473563638243327 ) ) ;
#18696=LINE ( 'NONE', #3565, #1842 ) ;
#18702=VECTOR ( 'NONE', #213, 1000.000000000000114 ) ;
#18703=DIRECTION ( 'NONE',  ( -0.000000000000000000, -1.000000000000000000, 0.000000000000000000 ) ) ;
#18704=FACE_OUTER_BOUND ( 'NONE', #10506, .T. ) ;
#18711=DIRECTION ( 'NONE',  ( 0.000000000000000000, -1.000000000000000000, -0.000000000000000000 ) ) ;
#18715=DIRECTION ( 'NONE',  ( -0.2064631973582987667, 0.000000000000000000, 0.9784543669157944601 ) ) ;
#18725=EDGE_CURVE ( 'NONE', #4163, #14616, #16954, .T. ) ;
#18734=VERTEX_POINT ( 'NONE', #7547 ) ;
#18748=EDGE_CURVE ( 'NONE', #1617, #4527, #16619, .T. ) ;
#18751=DIRECTION ( 'NONE',  ( 0.000000000000000000, 1.000000000000000000, 0.000000000000000000 ) ) ;
#18753=CARTESIAN_POINT ( 'NONE',  ( 38.82016491058538321, -9.531985000000000596, -14.75770094105646812 ) ) ;
#18754=AXIS2_PLACEMENT_3D ( 'NONE', #17936, #8296, #13301 ) ;
#18755=AXIS2_PLACEMENT_3D ( 'NONE', #1879, #8626, #15403 ) ;
#18757=LINE ( 'NONE', #11703, #21639 ) ;
#18758=DIRECTION ( 'NONE',  ( 0.000000000000000000, 1.000000000000000000, 0.000000000000000000 ) ) ;
#18759=FACE_OUTER_BOUND ( 'NONE', #13733, .T. ) ;
#18770=EDGE_LOOP ( 'NONE', ( #1620, #18228, #11137, #10023 ) ) ;
#18775=EDGE_CURVE ( 'NONE', #1384, #12537, #1006, .T. ) ;
#18778=DIRECTION ( 'NONE',  ( 0.000000000000000000, -1.000000000000000000, 0.000000000000000000 ) ) ;
#18784=DIRECTION ( 'NONE',  ( 0.000000000000000000, -1.000000000000000000, -0.000000000000000000 ) ) ;
#18786=VECTOR ( 'NONE', #10036, 1000.000000000000000 ) ;
#18789=CARTESIAN_POINT ( 'NONE',  ( 50.62387473582167274, 32.54502000000000095, -28.41576006634952734 ) ) ;
#18798=CARTESIAN_POINT ( 'NONE',  ( 42.79471501377724252, 0.000000000000000000, 5.049205022181460834 ) ) ;
#18799=EDGE_CURVE ( 'NONE', #1021, #7386, #12972, .T. ) ;
#18805=EDGE_CURVE ( 'NONE', #3173, #13394, #7078, .T. ) ;
#18810=CYLINDRICAL_SURFACE ( 'NONE', #6800, 0.7950199999999993938 ) ;
#18815=DIRECTION ( 'NONE',  ( 0.000000000000000000, 1.000000000000000000, 0.000000000000000000 ) ) ;
#18816=CARTESIAN_POINT ( 'NONE',  ( 38.60701496492545459, 34.52875999999999834, -26.94161103631838472 ) ) ;
#18820=CARTESIAN_POINT ( 'NONE',  ( 42.66304184606194383, -1.983739999999999837, -19.22597499813143784 ) ) ;
#18825=ORIENTED_EDGE ( 'NONE', *, *, #1948, .F. ) ;
#18827=EDGE_CURVE ( 'NONE', #2587, #10772, #19410, .T. ) ;
#18834=AXIS2_PLACEMENT_3D ( 'NONE', #18343, #3209, #10271 ) ;
#18838=DIRECTION ( 'NONE',  ( 0.000000000000000000, 1.000000000000000000, 0.000000000000000000 ) ) ;
#18858=EDGE_CURVE ( 'NONE', #4163, #15435, #17307, .T. ) ;
#18863=DIRECTION ( 'NONE',  ( 0.000000000000000000, 1.000000000000000000, 0.000000000000000000 ) ) ;
#18868=CARTESIAN_POINT ( 'NONE',  ( 55.14150854986954897, 38.88803500000000213, -23.45621182681304617 ) ) ;
#18869=ORIENTED_EDGE ( 'NONE', *, *, #9116, .T. ) ;
#18879=PLANE ( 'NONE',  #3604 ) ;
#18880=ORIENTED_EDGE ( 'NONE', *, *, #19135, .T. ) ;
#18890=CARTESIAN_POINT ( 'NONE',  ( 41.45112526417833010, 34.52875999999999834, 7.778260066349530710 ) ) ;
#18895=DIRECTION ( 'NONE',  ( -0.7421532822901579785, 0.000000000000000000, 0.6702301885068630005 ) ) ;
#18901=DIRECTION ( 'NONE',  ( 0.05085730733808393328, 0.000000000000000000, -0.9987059298363656357 ) ) ;
#18909=DIRECTION ( 'NONE',  ( -0.4987171968201928873, 0.000000000000000000, 0.8667647648559606566 ) ) ;
#18912=CARTESIAN_POINT ( 'NONE',  ( 38.96848998618624904, 40.07865999999999929, -3.934807454472129429 ) ) ;
#18917=CARTESIAN_POINT ( 'NONE',  ( 37.07154142533928365, -6.356984999999999886, -2.340318470350700508 ) ) ;
#18923=FACE_OUTER_BOUND ( 'NONE', #18202, .T. ) ;
#18924=CYLINDRICAL_SURFACE ( 'NONE', #20857, 30.16249999999999432 ) ;
#18926=CARTESIAN_POINT ( 'NONE',  ( 30.41963056417667488, 34.52875999999999834, -8.653862521447852174 ) ) ;
#18927=EDGE_CURVE ( 'NONE', #19208, #6484, #13145, .T. ) ;
#18930=CARTESIAN_POINT ( 'NONE',  ( 53.46798503507454825, -1.983739999999999837, 6.304111036318381878 ) ) ;
#18935=PLANE ( 'NONE',  #4757 ) ;
#18941=CARTESIAN_POINT ( 'NONE',  ( 39.62791084302666178, 0.000000000000000000, -24.65774797299118859 ) ) ;
#18942=EDGE_CURVE ( 'NONE', #11378, #17699, #12780, .T. ) ;
#18945=LINE ( 'NONE', #10340, #1065 ) ;
#18960=VERTEX_POINT ( 'NONE', #5189 ) ;
#18963=CARTESIAN_POINT ( 'NONE',  ( 39.11079947626275555, 32.54502000000000095, -27.65534212225540500 ) ) ;
#18964=ORIENTED_EDGE ( 'NONE', *, *, #19283, .T. ) ;
#18968=EDGE_CURVE ( 'NONE', #8481, #3974, #20422, .T. ) ;
#18970=CARTESIAN_POINT ( 'NONE',  ( 49.41195815393805901, 42.06303499999999929, -1.411525001868561224 ) ) ;
#18973=CARTESIAN_POINT ( 'NONE',  ( 38.78586790977451670, 38.88803500000000213, -5.374168024304903035 ) ) ;
#18974=CARTESIAN_POINT ( 'NONE',  ( 30.97944403357121956, 34.52875999999999834, -8.103300075789407586 ) ) ;
#18977=VERTEX_POINT ( 'NONE', #11938 ) ;
#18980=AXIS2_PLACEMENT_3D ( 'NONE', #325, #15281, #18566 ) ;
#18994=CARTESIAN_POINT ( 'NONE',  ( 38.55086098473930889, -7.409553547294740028, -4.428244049269694393 ) ) ;
#18997=EDGE_CURVE ( 'NONE', #2302, #8192, #3947, .T. ) ;
#19005=VERTEX_POINT ( 'NONE', #15284 ) ;
#19007=CARTESIAN_POINT ( 'NONE',  ( 39.07078961959606289, 34.52875999999999834, -27.14892015257980162 ) ) ;
#19012=AXIS2_PLACEMENT_3D ( 'NONE', #1233, #18572, #21452 ) ;
#19015=CARTESIAN_POINT ( 'NONE',  ( 61.09555596642878328, 0.000000000000000000, -12.53419992421059348 ) ) ;
#19020=DIRECTION ( 'NONE',  ( 0.000000000000000000, -1.000000000000000000, -0.000000000000000000 ) ) ;
#19021=CARTESIAN_POINT ( 'NONE',  ( 44.27024749654656688, -5.166360000000000063, -8.722764363618033201 ) ) ;
#19023=DIRECTION ( 'NONE',  ( -0.9987059298363656357, 0.000000000000000000, -0.05085730733808393328 ) ) ;
#19024=EDGE_CURVE ( 'NONE', #18977, #3969, #8179, .T. ) ;
#19034=ORIENTED_EDGE ( 'NONE', *, *, #12642, .F. ) ;
#19035=AXIS2_PLACEMENT_3D ( 'NONE', #3125, #19807, #19492 ) ;
#19039=ORIENTED_EDGE ( 'NONE', *, *, #18675, .F. ) ;
#19046=CIRCLE ( 'NONE', #15190, 0.5080000000000022276 ) ;
#19055=ORIENTED_EDGE ( 'NONE', *, *, #21483, .T. ) ;
#19063=AXIS2_PLACEMENT_3D ( 'NONE', #7033, #20505, #13927 ) ;
#19069=ORIENTED_EDGE ( 'NONE', *, *, #14252, .T. ) ;
#19075=CARTESIAN_POINT ( 'NONE',  ( 53.46798503507454825, 32.54502000000000095, 6.304111036318381878 ) ) ;
#19078=ADVANCED_FACE ( 'NONE', ( #18466 ), #15395, .T. ) ;
#19081=VECTOR ( 'NONE', #18703, 1000.000000000000000 ) ;
#19082=CARTESIAN_POINT ( 'NONE',  ( 39.93069333242032570, 38.88803500000010160, -3.008993689095761148 ) ) ;
#19085=FACE_OUTER_BOUND ( 'NONE', #20271, .T. ) ;
#19087=CARTESIAN_POINT ( 'NONE',  ( 36.73521423675246922, 34.52875999999999834, 2.413462327205186497 ) ) ;
#19090=ORIENTED_EDGE ( 'NONE', *, *, #17228, .F. ) ;
#19091=EDGE_LOOP ( 'NONE', ( #20513, #15771, #18340, #16982 ) ) ;
#19094=CARTESIAN_POINT ( 'NONE',  ( 34.72145145287101542, 37.11476346399999926, 0.5851394578805096947 ) ) ;
#19100=ORIENTED_EDGE ( 'NONE', *, *, #20903, .F. ) ;
#19101=EDGE_CURVE ( 'NONE', #6924, #8259, #8869, .T. ) ;
#19108=CARTESIAN_POINT ( 'NONE',  ( 52.44708915697334106, 34.52875999999999834, 4.020247972991190188 ) ) ;
#19109=DIRECTION ( 'NONE',  ( 0.9724402360367340181, 0.000000000000000000, -0.2331522835762512846 ) ) ;
#19114=VERTEX_POINT ( 'NONE', #18669 ) ;
#19116=CARTESIAN_POINT ( 'NONE',  ( 53.10651001381376091, 40.07865999999999929, -16.70269254552787075 ) ) ;
#19118=DIRECTION ( 'NONE',  ( -0.9987059298363656357, -0.000000000000000000, -0.05085730733808393328 ) ) ;
#19122=DIRECTION ( 'NONE',  ( 0.3928209820863022839, 0.000000000000000000, -0.9196149607486564515 ) ) ;
#19135=EDGE_CURVE ( 'NONE', #12957, #9108, #6860, .T. ) ;
#19136=AXIS2_PLACEMENT_3D ( 'NONE', #7999, #4897, #9760 ) ;
#19138=AXIS2_PLACEMENT_3D ( 'NONE', #5632, #330, #553 ) ;
#19145=CARTESIAN_POINT ( 'NONE',  ( 59.55063415577301811, -1.983739999999999837, -22.52230776719629191 ) ) ;
#19147=CARTESIAN_POINT ( 'NONE',  ( 37.51913901087312553, 42.06303499999999929, -14.58057485080488114 ) ) ;
#19148=CARTESIAN_POINT ( 'NONE',  ( 49.13030338002142372, 0.000000000000000000, -2.154981381712871791 ) ) ;
#19150=CARTESIAN_POINT ( 'NONE',  ( 31.04121718565060206, 34.52875999999999834, -8.720124554639784975 ) ) ;
#19155=ORIENTED_EDGE ( 'NONE', *, *, #5838, .T. ) ;
#19163=AXIS2_PLACEMENT_3D ( 'NONE', #16580, #5947, #11155 ) ;
#19165=EDGE_CURVE ( 'NONE', #8304, #13851, #2885, .T. ) ;
#19174=CARTESIAN_POINT ( 'NONE',  ( 39.42154620619643879, -5.166360000000000063, -4.343957374020580353 ) ) ;
#19175=VERTEX_POINT ( 'NONE', #7298 ) ;
#19177=CARTESIAN_POINT ( 'NONE',  ( 52.91086381164393515, 37.11476346399999926, 3.812938856729753301 ) ) ;
#19178=ORIENTED_EDGE ( 'NONE', *, *, #9791, .F. ) ;
#19188=CARTESIAN_POINT ( 'NONE',  ( 39.48015564263409516, -5.405895081254803891, -3.409410579613285197 ) ) ;
#19189=ORIENTED_EDGE ( 'NONE', *, *, #4405, .F. ) ;
#19192=CIRCLE ( 'NONE', #14266, 0.5080000000000013394 ) ;
#19195=ORIENTED_EDGE ( 'NONE', *, *, #19670, .T. ) ;
#19196=DIRECTION ( 'NONE',  ( 0.000000000000000000, 1.000000000000000000, 0.000000000000000000 ) ) ;
#19200=CARTESIAN_POINT ( 'NONE',  ( 38.94885947252247860, -7.547248457916676756, -3.956611957470116625 ) ) ;
#19201=VERTEX_POINT ( 'NONE', #5749 ) ;
#19208=VERTEX_POINT ( 'NONE', #19116 ) ;
#19210=VERTEX_POINT ( 'NONE', #8724 ) ;
#19216=ORIENTED_EDGE ( 'NONE', *, *, #360, .F. ) ;
#19218=AXIS2_PLACEMENT_3D ( 'NONE', #8043, #14816, #7720 ) ;
#19220=LINE ( 'NONE', #1976, #4033 ) ;
#19227=AXIS2_PLACEMENT_3D ( 'NONE', #21225, #7745, #16567 ) ;
#19232=FACE_OUTER_BOUND ( 'NONE', #12673, .T. ) ;
#19235=FACE_OUTER_BOUND ( 'NONE', #20300, .T. ) ;
#19238=ORIENTED_EDGE ( 'NONE', *, *, #14997, .F. ) ;
#19241=DIRECTION ( 'NONE',  ( -0.000000000000000000, -1.000000000000000000, 0.000000000000000000 ) ) ;
#19247=FACE_OUTER_BOUND ( 'NONE', #20552, .T. ) ;
#19248=EDGE_CURVE ( 'NONE', #723, #10564, #17003, .T. ) ;
#19249=DIRECTION ( 'NONE',  ( 0.05085730733808139364, 0.000000000000000000, -0.9987059298363658577 ) ) ;
#19261=ORIENTED_EDGE ( 'NONE', *, *, #6111, .F. ) ;
#19263=CARTESIAN_POINT ( 'NONE',  ( 59.55063415577301811, 32.54502000000000095, -22.52230776719629191 ) ) ;
#19264=EDGE_CURVE ( 'NONE', #8553, #16810, #13859, .T. ) ;
#19265=DIRECTION ( 'NONE',  ( 0.000000000000000000, 1.000000000000000000, 0.000000000000000000 ) ) ;
#19267=ORIENTED_EDGE ( 'NONE', *, *, #4646, .F. ) ;
#19279=LINE ( 'NONE', #15777, #21335 ) ;
#19281=EDGE_CURVE ( 'NONE', #3095, #16730, #5630, .T. ) ;
#19283=EDGE_CURVE ( 'NONE', #17699, #11223, #9582, .T. ) ;
#19285=ORIENTED_EDGE ( 'NONE', *, *, #4953, .T. ) ;
#19287=DIRECTION ( 'NONE',  ( 0.000000000000000000, -1.000000000000000000, -0.000000000000000000 ) ) ;
#19294=EDGE_LOOP ( 'NONE', ( #10129, #5753, #9820, #21279, #10040 ) ) ;
#19296=CYLINDRICAL_SURFACE ( 'NONE', #13032, 0.7950199999999993938 ) ;
#19302=CARTESIAN_POINT ( 'NONE',  ( 46.03750000000000142, 42.06303499999999929, -10.31874999999999964 ) ) ;
#19303=CIRCLE ( 'NONE', #5522, 30.16249999999998721 ) ;
#19309=FACE_OUTER_BOUND ( 'NONE', #18005, .T. ) ;
#19311=VERTEX_POINT ( 'NONE', #14283 ) ;
#19318=EDGE_LOOP ( 'NONE', ( #19238, #20805, #3202, #935 ) ) ;
#19319=CIRCLE ( 'NONE', #15814, 1.190624999999999378 ) ;
#19330=CARTESIAN_POINT ( 'NONE',  ( 32.52436584422698473, 34.52875999999999834, 1.884807767196291284 ) ) ;
#19340=ORIENTED_EDGE ( 'NONE', *, *, #21551, .F. ) ;
#19341=LINE ( 'NONE', #9500, #12759 ) ;
#19355=LINE ( 'NONE', #18917, #6810 ) ;
#19356=EDGE_CURVE ( 'NONE', #10995, #12131, #12074, .T. ) ;
#19358=EDGE_CURVE ( 'NONE', #11223, #20800, #3595, .T. ) ;
#19361=CARTESIAN_POINT ( 'NONE',  ( 50.52547294529469468, 38.88803500000000213, -18.64987929725020521 ) ) ;
#19365=CARTESIAN_POINT ( 'NONE',  ( 53.46798503507454825, 32.54502000000000095, 6.304111036318381878 ) ) ;
#19371=DIRECTION ( 'NONE',  ( 0.05085730733808139364, 0.000000000000000000, -0.9987059298363658577 ) ) ;
#19372=ORIENTED_EDGE ( 'NONE', *, *, #14369, .F. ) ;
#19384=ADVANCED_FACE ( 'NONE', ( #14717 ), #14610, .T. ) ;
#19386=CARTESIAN_POINT ( 'NONE',  ( 53.77854886916050958, -7.114547009363026753, -15.86998015261754880 ) ) ;
#19399=CIRCLE ( 'NONE', #13788, 0.5079999999999995630 ) ;
#19402=ADVANCED_FACE ( 'NONE', ( #21426 ), #13052, .F. ) ;
#19406=DIRECTION ( 'NONE',  ( -0.8943161143440100380, 0.000000000000000000, -0.4474356798743607255 ) ) ;
#19410=CIRCLE ( 'NONE', #16275, 30.16249999999999076 ) ;
#19411=FACE_OUTER_BOUND ( 'NONE', #21660, .T. ) ;
#19416=VERTEX_POINT ( 'NONE', #19330 ) ;
#19422=ORIENTED_EDGE ( 'NONE', *, *, #12703, .F. ) ;
#19426=ORIENTED_EDGE ( 'NONE', *, *, #8325, .T. ) ;
#19427=AXIS2_PLACEMENT_3D ( 'NONE', #2458, #8974, #10858 ) ;
#19435=VERTEX_POINT ( 'NONE', #2652 ) ;
#19437=CARTESIAN_POINT ( 'NONE',  ( 39.47397446732132664, 38.88803500000000213, 2.793231391354656701 ) ) ;
#19448=AXIS2_PLACEMENT_3D ( 'NONE', #19150, #2351, #7232 ) ;
#19455=EDGE_CURVE ( 'NONE', #15606, #19114, #17688, .T. ) ;
#19460=AXIS2_PLACEMENT_3D ( 'NONE', #2206, #551, #15608 ) ;
#19462=CARTESIAN_POINT ( 'NONE',  ( 52.91474337680157447, -7.548011381845581624, -16.50491988134626808 ) ) ;
#19464=DIRECTION ( 'NONE',  ( 0.1060008583745224581, 0.000000000000000000, 0.9943660382494288186 ) ) ;
#19467=LINE ( 'NONE', #19145, #17044 ) ;
#19469=DIRECTION ( 'NONE',  ( -0.3542738219355860418, 0.000000000000000000, -0.9351417320872557060 ) ) ;
#19470=DIRECTION ( 'NONE',  ( -0.7421532822901579785, -0.000000000000000000, 0.6702301885068630005 ) ) ;
#19472=ORIENTED_EDGE ( 'NONE', *, *, #19953, .T. ) ;
#19475=AXIS2_PLACEMENT_3D ( 'NONE', #2547, #16374, #7628 ) ;
#19485=ORIENTED_EDGE ( 'NONE', *, *, #18290, .F. ) ;
#19491=AXIS2_PLACEMENT_3D ( 'NONE', #20295, #13478, #15043 ) ;
#19492=DIRECTION ( 'NONE',  ( -0.9724402360367336851, 0.000000000000000000, 0.2331522835762537549 ) ) ;
#19499=CARTESIAN_POINT ( 'NONE',  ( 53.91018755822011599, -6.683201455308112493, -15.68072631912343518 ) ) ;
#19505=EDGE_CURVE ( 'NONE', #11144, #3974, #11030, .T. ) ;
#19508=ORIENTED_EDGE ( 'NONE', *, *, #17190, .F. ) ;
#19521=VECTOR ( 'NONE', #14383, 1000.000000000000000 ) ;
#19531=VERTEX_POINT ( 'NONE', #15042 ) ;
#19543=ORIENTED_EDGE ( 'NONE', *, *, #20692, .F. ) ;
#19548=ORIENTED_EDGE ( 'NONE', *, *, #20068, .F. ) ;
#19549=PLANE ( 'NONE',  #1822 ) ;
#19551=CARTESIAN_POINT ( 'NONE',  ( 38.96848998618624904, -5.166360000000000063, -3.934807454472129429 ) ) ;
#19558=DIRECTION ( 'NONE',  ( -0.6702301885068638887, 0.000000000000000000, -0.7421532822901570903 ) ) ;
#19560=ORIENTED_EDGE ( 'NONE', *, *, #498, .F. ) ;
#19565=FACE_BOUND ( 'NONE', #15675, .T. ) ;
#19568=ORIENTED_EDGE ( 'NONE', *, *, #9263, .T. ) ;
#19579=DIRECTION ( 'NONE',  ( 0.5222415575336524229, 0.000000000000000000, 0.8527976052879281399 ) ) ;
#19582=CARTESIAN_POINT ( 'NONE',  ( 34.38097451710952868, 0.000000000000000000, 0.2081255904771098786 ) ) ;
#19584=CARTESIAN_POINT ( 'NONE',  ( 42.94469661997857912, 42.06303499999999929, -18.48251861828712705 ) ) ;
#19587=ORIENTED_EDGE ( 'NONE', *, *, #11806, .T. ) ;
#19592=CARTESIAN_POINT ( 'NONE',  ( 27.93207353965470574, 34.52875999999999834, -8.388685343514779902 ) ) ;
#19598=LINE ( 'NONE', #4464, #709 ) ;
#19599=LINE ( 'NONE', #4357, #147 ) ;
#19608=VERTEX_POINT ( 'NONE', #18230 ) ;
#19611=AXIS2_PLACEMENT_3D ( 'NONE', #20737, #17210, #5594 ) ;
#19618=CARTESIAN_POINT ( 'NONE',  ( 41.45112526417833010, 32.54502000000000095, 7.778260066349530710 ) ) ;
#19620=ORIENTED_EDGE ( 'NONE', *, *, #137, .T. ) ;
#19630=EDGE_CURVE ( 'NONE', #20092, #4911, #1488, .T. ) ;
#19635=DIRECTION ( 'NONE',  ( 0.000000000000000000, 1.000000000000000000, 0.000000000000000000 ) ) ;
#19637=DIRECTION ( 'NONE',  ( 0.000000000000000000, 1.000000000000000000, 0.000000000000000000 ) ) ;
#19640=ORIENTED_EDGE ( 'NONE', *, *, #17069, .F. ) ;
#19643=CIRCLE ( 'NONE', #18245, 0.5079999999999993410 ) ;
#19644=ORIENTED_EDGE ( 'NONE', *, *, #1169, .T. ) ;
#19646=ADVANCED_FACE ( 'NONE', ( #18441 ), #11486, .F. ) ;
#19650=DIRECTION ( 'NONE',  ( 0.000000000000000000, 1.000000000000000000, 0.000000000000000000 ) ) ;
#19652=ORIENTED_EDGE ( 'NONE', *, *, #8436, .T. ) ;
#19653=EDGE_CURVE ( 'NONE', #3095, #12537, #15143, .T. ) ;
#19655=DIRECTION ( 'NONE',  ( -0.3542738219355896501, 0.000000000000000000, -0.9351417320872542627 ) ) ;
#19658=ORIENTED_EDGE ( 'NONE', *, *, #19630, .F. ) ;
#19665=ORIENTED_EDGE ( 'NONE', *, *, #21255, .T. ) ;
#19667=CYLINDRICAL_SURFACE ( 'NONE', #17338, 0.5079999999999995630 ) ;
#19670=EDGE_CURVE ( 'NONE', #2248, #7998, #11722, .T. ) ;
#19678=FACE_OUTER_BOUND ( 'NONE', #17547, .T. ) ;
#19680=DIRECTION ( 'NONE',  ( -0.2227372614607790735, 0.000000000000000000, -0.9748785115884710528 ) ) ;
#19681=CARTESIAN_POINT ( 'NONE',  ( 53.92979111630293687, -6.275737754352774367, -15.65141968183263899 ) ) ;
#19684=LINE ( 'NONE', #6205, #2169 ) ;
#19687=EDGE_LOOP ( 'NONE', ( #14054, #1312, #20053, #3286 ) ) ;
#19688=LINE ( 'NONE', #2689, #1806 ) ;
#19696=EDGE_CURVE ( 'NONE', #8373, #8830, #3191, .T. ) ;
#19701=AXIS2_PLACEMENT_3D ( 'NONE', #2612, #11222, #7795 ) ;
#19702=DIRECTION ( 'NONE',  ( 0.000000000000000000, 1.000000000000000000, 0.000000000000000000 ) ) ;
#19704=CARTESIAN_POINT ( 'NONE',  ( 53.08681243024872742, 40.07829845791615497, -16.72443647849243575 ) ) ;
#19707=ORIENTED_EDGE ( 'NONE', *, *, #20541, .F. ) ;
#19710=CYLINDRICAL_SURFACE ( 'NONE', #9057, 1.190625000000000711 ) ;
#19724=EDGE_LOOP ( 'NONE', ( #6139, #20057, #11576, #11199 ) ) ;
#19730=( LENGTH_UNIT ( ) NAMED_UNIT ( * ) SI_UNIT ( .MILLI., .METRE. ) );
#19740=ORIENTED_EDGE ( 'NONE', *, *, #3410, .F. ) ;
#19743=ORIENTED_EDGE ( 'NONE', *, *, #4072, .T. ) ;
#19751=DIRECTION ( 'NONE',  ( -0.9129422336036123742, -0.000000000000000000, 0.4080888115384289083 ) ) ;
#19753=CARTESIAN_POINT ( 'NONE',  ( 39.11540848302676210, 37.69142280624949848, -3.773741628647232726 ) ) ;
#19769=ADVANCED_FACE ( 'NONE', ( #8695 ), #15474, .T. ) ;
#19771=CARTESIAN_POINT ( 'NONE',  ( 39.00487391864218267, 37.69864044684034354, -3.894748490052650780 ) ) ;
#19773=AXIS2_PLACEMENT_3D ( 'NONE', #10882, #9436, #2483 ) ;
#19777=AXIS2_PLACEMENT_3D ( 'NONE', #7847, #780, #9284 ) ;
#19787=CARTESIAN_POINT ( 'NONE',  ( 36.80301088673436283, 34.52875999999999834, -23.10021947667301134 ) ) ;
#19790=ORIENTED_EDGE ( 'NONE', *, *, #12304, .T. ) ;
#19797=ADVANCED_FACE ( 'NONE', ( #13932 ), #2059, .T. ) ;
#19807=DIRECTION ( 'NONE',  ( 0.000000000000000000, 1.000000000000000000, 0.000000000000000000 ) ) ;
#19822=ORIENTED_EDGE ( 'NONE', *, *, #18997, .F. ) ;
#19825=ORIENTED_EDGE ( 'NONE', *, *, #12085, .T. ) ;
#19829=CARTESIAN_POINT ( 'NONE',  ( 52.19854938732527216, 38.88803500000000213, -17.58284632693144189 ) ) ;
#19835=AXIS2_PLACEMENT_3D ( 'NONE', #6506, #3081, #4624 ) ;
#19837=DIRECTION ( 'NONE',  ( -0.9129422336036127072, 0.000000000000000000, 0.4080888115384278536 ) ) ;
#19841=CIRCLE ( 'NONE', #2908, 0.5080000000000007843 ) ;
#19849=FACE_OUTER_BOUND ( 'NONE', #8466, .T. ) ;
#19859=VERTEX_POINT ( 'NONE', #18974 ) ;
#19876=CARTESIAN_POINT ( 'NONE',  ( 53.76169727759691597, 38.28855596976028863, -15.89243902784262197 ) ) ;
#19884=DIRECTION ( 'NONE',  ( 0.7421532822901579785, 0.000000000000000000, -0.6702301885068630005 ) ) ;
#19888=AXIS2_PLACEMENT_3D ( 'NONE', #15133, #3298, #16781 ) ;
#19901=CARTESIAN_POINT ( 'NONE',  ( 39.58386072796550081, 38.88803500000000213, -4.490541772578183100 ) ) ;
#19904=ORIENTED_EDGE ( 'NONE', *, *, #16755, .F. ) ;
#19907=EDGE_CURVE ( 'NONE', #18598, #14787, #13160, .T. ) ;
#19909=CARTESIAN_POINT ( 'NONE',  ( 61.65536943582333151, 32.54502000000000095, -11.98363747855214712 ) ) ;
#19917=DIRECTION ( 'NONE',  ( 0.000000000000000000, -1.000000000000000000, -0.000000000000000000 ) ) ;
#19924=EDGE_CURVE ( 'NONE', #1990, #8373, #21597, .T. ) ;
#19925=DIRECTION ( 'NONE',  ( 0.9943660382494290406, 0.000000000000000000, -0.1060008583745199739 ) ) ;
#19927=DIRECTION ( 'NONE',  ( 0.000000000000000000, 0.000000000000000000, -1.000000000000000000 ) ) ;
#19928=DIRECTION ( 'NONE',  ( 0.000000000000000000, -1.000000000000000000, -0.000000000000000000 ) ) ;
#19929=CARTESIAN_POINT ( 'NONE',  ( 52.65345379380355695, 40.07865999999999929, -16.29354262597941982 ) ) ;
#19933=DIRECTION ( 'NONE',  ( -0.9959941601142527912, 0.000000000000000000, -0.08941830359777887260 ) ) ;
#19934=CARTESIAN_POINT ( 'NONE',  ( 46.03750000000000142, 34.52875999999999834, -10.31874999999999964 ) ) ;
#19937=CARTESIAN_POINT ( 'NONE',  ( 49.41195815393805901, 0.000000000000000000, -1.411525001868561224 ) ) ;
#19941=DIRECTION ( 'NONE',  ( 0.000000000000000000, 1.000000000000000000, 0.000000000000000000 ) ) ;
#19942=ORIENTED_EDGE ( 'NONE', *, *, #8101, .F. ) ;
#19945=EDGE_LOOP ( 'NONE', ( #5721, #12489 ) ) ;
#19953=EDGE_CURVE ( 'NONE', #20253, #18266, #459, .T. ) ;
#19956=B_SPLINE_CURVE_WITH_KNOTS ( 'NONE', 3,
 ( #9481, #19753, #4516, #4625, #21091, #1081, #21199, #12830, #5941, #16043, #9590, #12707 ),
 .UNSPECIFIED., .F., .F.,
 ( 4, 2, 2, 2, 2, 4 ),
 ( 0.001626748932157576297, 0.002113374744101624396, 0.002356687650073656035, 0.002600000556045687240, 0.003086626367989763961, 0.003573252179933841116 ),
 .UNSPECIFIED. ) ;
#19960=DIRECTION ( 'NONE',  ( -0.000000000000000000, -1.000000000000000000, 0.000000000000000000 ) ) ;
#19961=ORIENTED_EDGE ( 'NONE', *, *, #18533, .F. ) ;
#19962=ORIENTED_EDGE ( 'NONE', *, *, #14153, .F. ) ;
#19963=CARTESIAN_POINT ( 'NONE',  ( 52.96420052373725440, 34.52875999999999834, 7.017842122255405712 ) ) ;
#19970=CARTESIAN_POINT ( 'NONE',  ( 32.42378190387104553, 0.000000000000000000, -18.15178106273469183 ) ) ;
#19971=EDGE_LOOP ( 'NONE', ( #16874, #3467, #20426, #18103 ) ) ;
#19977=CARTESIAN_POINT ( 'NONE',  ( 38.54095024924464497, 38.88803500000000213, -2.295677052105690841 ) ) ;
#19980=LINE ( 'NONE', #8475, #4700 ) ;
#19982=CYLINDRICAL_SURFACE ( 'NONE', #12807, 0.5080000000000000071 ) ;
#19990=DIRECTION ( 'NONE',  ( -0.6702301885068628895, 0.000000000000000000, -0.7421532822901579785 ) ) ;
#19994=CARTESIAN_POINT ( 'NONE',  ( 59.52193197173441774, 34.52875999999999834, -3.260183413611184911 ) ) ;
#19998=DIRECTION ( 'NONE',  ( -0.7421532822901579785, 0.000000000000000000, 0.6702301885068628895 ) ) ;
#20002=DIRECTION ( 'NONE',  ( 0.000000000000000000, 1.000000000000000000, 0.000000000000000000 ) ) ;
#20005=CARTESIAN_POINT ( 'NONE',  ( 42.79471501377724252, 0.000000000000000000, 5.049205022181460834 ) ) ;
#20006=ORIENTED_EDGE ( 'NONE', *, *, #16862, .T. ) ;
#20018=EDGE_CURVE ( 'NONE', #7959, #18042, #3136, .T. ) ;
#20023=DIRECTION ( 'NONE',  ( 0.000000000000000000, 1.000000000000000000, -0.000000000000000000 ) ) ;
#20039=DIRECTION ( 'NONE',  ( -0.000000000000000000, -1.000000000000000000, 0.000000000000000000 ) ) ;
#20042=EDGE_CURVE ( 'NONE', #16209, #10716, #434, .T. ) ;
#20047=ADVANCED_FACE ( 'NONE', ( #16210 ), #13003, .F. ) ;
#20053=ORIENTED_EDGE ( 'NONE', *, *, #210, .F. ) ;
#20056=CARTESIAN_POINT ( 'NONE',  ( 38.96520571134880129, -5.166360000000000952, -3.938444168234590315 ) ) ;
#20057=ORIENTED_EDGE ( 'NONE', *, *, #12642, .T. ) ;
#20060=CARTESIAN_POINT ( 'NONE',  ( 61.83151161312219557, -1.983739999999999837, -0.3645647634491749334 ) ) ;
#20063=EDGE_LOOP ( 'NONE', ( #4414, #13335, #18492, #56 ) ) ;
#20066=VERTEX_POINT ( 'NONE', #18816 ) ;
#20067=EDGE_CURVE ( 'NONE', #5196, #19435, #16840, .T. ) ;
#20068=EDGE_CURVE ( 'NONE', #14783, #8133, #8533, .T. ) ;
#20071=AXIS2_PLACEMENT_3D ( 'NONE', #12206, #20249, #15427 ) ;
#20073=ORIENTED_EDGE ( 'NONE', *, *, #9263, .F. ) ;
#20079=ADVANCED_FACE ( 'NONE', ( #13877, #8420 ), #15314, .T. ) ;
#20080=ORIENTED_EDGE ( 'NONE', *, *, #14472, .T. ) ;
#20085=CARTESIAN_POINT ( 'NONE',  ( 53.49555360346280963, 37.84815426416190576, -16.24526707472953291 ) ) ;
#20089=FACE_OUTER_BOUND ( 'NONE', #18421, .T. ) ;
#20090=ORIENTED_EDGE ( 'NONE', *, *, #18624, .F. ) ;
#20092=VERTEX_POINT ( 'NONE', #6988 ) ;
#20093=ADVANCED_FACE ( 'NONE', ( #18704 ), #24, .T. ) ;
#20097=DIRECTION ( 'NONE',  ( 0.000000000000000000, -1.000000000000000000, -0.000000000000000000 ) ) ;
#20099=LINE ( 'NONE', #15496, #170 ) ;
#20101=CIRCLE ( 'NONE', #13131, 30.16249999999999787 ) ;
#20102=ORIENTED_EDGE ( 'NONE', *, *, #3559, .T. ) ;
#20107=CARTESIAN_POINT ( 'NONE',  ( 39.62791084302666178, 0.000000000000000000, -24.65774797299118859 ) ) ;
#20112=STYLED_ITEM ( 'NONE', ( #16655 ), #13288 ) ;
#20113=ADVANCED_FACE ( 'NONE', ( #17055 ), #1901, .F. ) ;
#20115=DIRECTION ( 'NONE',  ( 0.000000000000000000, 1.000000000000000000, -0.000000000000000000 ) ) ;
#20130=AXIS2_PLACEMENT_3D ( 'NONE', #3373, #16852, #8430 ) ;
#20132=ORIENTED_EDGE ( 'NONE', *, *, #8715, .T. ) ;
#20135=DIRECTION ( 'NONE',  ( 0.05085730733808393328, 0.000000000000000000, -0.9987059298363656357 ) ) ;
#20138=CARTESIAN_POINT ( 'NONE',  ( 52.96420052373725440, -1.983739999999999837, 7.017842122255405712 ) ) ;
#20147=B_SPLINE_CURVE_WITH_KNOTS ( 'NONE', 3,
 ( #4258, #2488, #830, #10887, #5904, #504, #5694, #934, #4149, #20825, #14336, #3822 ),
 .UNSPECIFIED., .F., .F.,
 ( 4, 2, 2, 2, 2, 4 ),
 ( 0.0005892739765683242207, 0.001065175039931907409, 0.001303125571613693908, 0.001541076103295480624, 0.002016977166659053404, 0.002492878230022626835 ),
 .UNSPECIFIED. ) ;
#20149=AXIS2_PLACEMENT_3D ( 'NONE', #6479, #5030, #13242 ) ;
#20151=ORIENTED_EDGE ( 'NONE', *, *, #36, .T. ) ;
#20162=CYLINDRICAL_SURFACE ( 'NONE', #6410, 30.16250000000000142 ) ;
#20166=CIRCLE ( 'NONE', #16327, 0.5080000000000011173 ) ;
#20168=DIRECTION ( 'NONE',  ( 0.4987171968201936645, 0.000000000000000000, -0.8667647648559603235 ) ) ;
#20177=ORIENTED_EDGE ( 'NONE', *, *, #16803, .T. ) ;
#20180=DIRECTION ( 'NONE',  ( -0.9129422336036123742, -0.000000000000000000, 0.4080888115384289083 ) ) ;
#20182=CIRCLE ( 'NONE', #2550, 1.190625000000000711 ) ;
#20186=DIRECTION ( 'NONE',  ( -0.9987059298363656357, 0.000000000000000000, -0.05085730733808393328 ) ) ;
#20187=EDGE_CURVE ( 'NONE', #1735, #21211, #11415, .T. ) ;
#20188=CARTESIAN_POINT ( 'NONE',  ( 39.58386072796507449, 40.07865999999999929, -4.490541772578644064 ) ) ;
#20192=CIRCLE ( 'NONE', #14590, 0.5079999999999985638 ) ;
#20194=CARTESIAN_POINT ( 'NONE',  ( 47.00675968526203263, -6.356984999999999886, -12.79836188810915232 ) ) ;
#20197=DIRECTION ( 'NONE',  ( 0.9943660382494290406, 0.000000000000000000, -0.1060008583745199739 ) ) ;
#20203=CARTESIAN_POINT ( 'NONE',  ( 44.27024749654656688, -6.356984999999999886, -8.722764363618033201 ) ) ;
#20205=AXIS2_PLACEMENT_3D ( 'NONE', #13869, #3899, #5318 ) ;
#20208=ORIENTED_EDGE ( 'NONE', *, *, #8273, .F. ) ;
#20217=ORIENTED_EDGE ( 'NONE', *, *, #7748, .T. ) ;
#20220=CARTESIAN_POINT ( 'NONE',  ( 53.63564901804143403, -5.379280274696189856, -16.06402915141540433 ) ) ;
#20224=AXIS2_PLACEMENT_3D ( 'NONE', #1621, #13264, #10030 ) ;
#20227=ORIENTED_EDGE ( 'NONE', *, *, #16189, .F. ) ;
#20241=CARTESIAN_POINT ( 'NONE',  ( 32.18388890846549799, -1.983739999999999837, 1.507793899792891468 ) ) ;
#20249=DIRECTION ( 'NONE',  ( 0.05085730733808393328, 0.000000000000000000, -0.9987059298363656357 ) ) ;
#20251=CARTESIAN_POINT ( 'NONE',  ( 30.47347900023190803, 34.52875999999999834, -8.148724574017967015 ) ) ;
#20253=VERTEX_POINT ( 'NONE', #16749 ) ;
#20258=AXIS2_PLACEMENT_3D ( 'NONE', #4035, #16099, #824 ) ;
#20267=ORIENTED_EDGE ( 'NONE', *, *, #1060, .F. ) ;
#20271=EDGE_LOOP ( 'NONE', ( #9474, #1398, #8254, #3949 ) ) ;
#20280=ORIENTED_EDGE ( 'NONE', *, *, #11755, .F. ) ;
#20291=FACE_OUTER_BOUND ( 'NONE', #621, .T. ) ;
#20293=CARTESIAN_POINT ( 'NONE',  ( 53.08681243026497043, 37.69777154208443193, -16.72443647847455850 ) ) ;
#20295=CARTESIAN_POINT ( 'NONE',  ( 46.03750000000000142, 42.06303499999999929, -10.31874999999999964 ) ) ;
#20300=EDGE_LOOP ( 'NONE', ( #8276, #16670, #16324, #1881, #5678, #9220, #1293, #1726, #20584, #11509, #9216, #924, #14151, #3315, #18474, #5143, #11925, #7713, #11124, #19155, #20978, #16058, #2440, #5410, #17966, #3931, #3308, #7924, #4102, #8459, #16556, #557, #3499, #20553, #5198, #5581, #8357, #16329, #15885, #10054 ) ) ;
#20307=FACE_OUTER_BOUND ( 'NONE', #6363, .T. ) ;
#20311=EDGE_CURVE ( 'NONE', #13568, #10812, #173, .T. ) ;
#20314=FACE_OUTER_BOUND ( 'NONE', #19091, .T. ) ;
#20317=VERTEX_POINT ( 'NONE', #1828 ) ;
#20322=VERTEX_POINT ( 'NONE', #13678 ) ;
#20337=VECTOR ( 'NONE', #3575, 1000.000000000000114 ) ;
#20344=DIRECTION ( 'NONE',  ( 0.7421532822901579785, 0.000000000000000000, -0.6702301885068630005 ) ) ;
#20349=CARTESIAN_POINT ( 'NONE',  ( 42.66304184606194383, 34.52875999999999834, -19.22597499813143784 ) ) ;
#20350=EDGE_LOOP ( 'NONE', ( #14424, #14587, #7523, #4273 ) ) ;
#20356=EDGE_LOOP ( 'NONE', ( #19261, #15449, #10014, #20864, #12700 ) ) ;
#20369=AXIS2_PLACEMENT_3D ( 'NONE', #11728, #1226, #6417 ) ;
#20370=DIRECTION ( 'NONE',  ( 0.000000000000000000, 1.000000000000000000, -0.000000000000000000 ) ) ;
#20372=DIRECTION ( 'NONE',  ( -0.07875956036501312318, 0.000000000000000000, 0.9968936410927243807 ) ) ;
#20373=VERTEX_POINT ( 'NONE', #5363 ) ;
#20376=ORIENTED_EDGE ( 'NONE', *, *, #3156, .F. ) ;
#20384=CARTESIAN_POINT ( 'NONE',  ( 54.55586098912687731, 34.52876000000000545, -6.056925149195119040 ) ) ;
#20386=ORIENTED_EDGE ( 'NONE', *, *, #17626, .F. ) ;
#20387=CARTESIAN_POINT ( 'NONE',  ( 30.47347900023190803, -1.983739999999999837, -8.148724574017967015 ) ) ;
#20392=LINE ( 'NONE', #12017, #2478 ) ;
#20395=CARTESIAN_POINT ( 'NONE',  ( 52.65345379380397617, 38.88803500000000213, -16.29354262597895087 ) ) ;
#20398=DIRECTION ( 'NONE',  ( 0.000000000000000000, 1.000000000000000000, 0.000000000000000000 ) ) ;
#20402=ORIENTED_EDGE ( 'NONE', *, *, #19505, .F. ) ;
#20403=ORIENTED_EDGE ( 'NONE', *, *, #12938, .F. ) ;
#20411=EDGE_LOOP ( 'NONE', ( #20090, #4169, #5416, #10794, #7529, #14574 ) ) ;
#20419=DIRECTION ( 'NONE',  ( 0.000000000000000000, -1.000000000000000000, -0.000000000000000000 ) ) ;
#20422=LINE ( 'NONE', #13300, #3234 ) ;
#20423=CARTESIAN_POINT ( 'NONE',  ( 59.55063415577301811, 34.52875999999999834, -22.52230776719629191 ) ) ;
#20426=ORIENTED_EDGE ( 'NONE', *, *, #1951, .T. ) ;
#20428=VECTOR ( 'NONE', #19287, 1000.000000000000000 ) ;
#20436=CARTESIAN_POINT ( 'NONE',  ( 39.26920185518109463, -7.547609999999999708, -4.208102635185587914 ) ) ;
#20437=ADVANCED_FACE ( 'NONE', ( #16321 ), #14342, .T. ) ;
#20440=CARTESIAN_POINT ( 'NONE',  ( 43.29176983217143260, 0.000000000000000000, 5.154088326438659884 ) ) ;
#20445=DIRECTION ( 'NONE',  ( 0.000000000000000000, 1.000000000000000000, 0.000000000000000000 ) ) ;
#20449=AXIS2_PLACEMENT_3D ( 'NONE', #5969, #2677, #7966 ) ;
#20454=AXIS2_PLACEMENT_3D ( 'NONE', #15997, #4145, #10783 ) ;
#20456=CARTESIAN_POINT ( 'NONE',  ( 61.81956123787853130, 0.000000000000000000, -1.238102447480925239 ) ) ;
#20457=EDGE_CURVE ( 'NONE', #1126, #8118, #15385, .T. ) ;
#20458=CARTESIAN_POINT ( 'NONE',  ( 31.05388211198297554, 34.52875999999999834, -15.23127950648024331 ) ) ;
#20461=ORIENTED_EDGE ( 'NONE', *, *, #137, .F. ) ;
#20463=CIRCLE ( 'NONE', #18652, 30.16250000000000497 ) ;
#20466=CARTESIAN_POINT ( 'NONE',  ( 31.05388211198297554, 34.52875999999999834, -15.23127950648024331 ) ) ;
#20475=ORIENTED_EDGE ( 'NONE', *, *, #12609, .T. ) ;
#20481=CARTESIAN_POINT ( 'NONE',  ( 31.05388211198297554, 0.000000000000000000, -15.23127950648024331 ) ) ;
#20491=CARTESIAN_POINT ( 'NONE',  ( 35.15748561355322011, 0.000000000000000000, 0.3244898641346534163 ) ) ;
#20498=DIRECTION ( 'NONE',  ( 0.7421532822901579785, 0.000000000000000000, -0.6702301885068628895 ) ) ;
#20500=ORIENTED_EDGE ( 'NONE', *, *, #14517, .T. ) ;
#20502=ORIENTED_EDGE ( 'NONE', *, *, #9761, .F. ) ;
#20503=AXIS2_PLACEMENT_3D ( 'NONE', #3411, #15257, #10143 ) ;
#20505=DIRECTION ( 'NONE',  ( 0.000000000000000000, 1.000000000000000000, 0.000000000000000000 ) ) ;
#20506=AXIS2_PLACEMENT_3D ( 'NONE', #20693, #809, #13882 ) ;
#20513=ORIENTED_EDGE ( 'NONE', *, *, #6053, .T. ) ;
#20519=ORIENTED_EDGE ( 'NONE', *, *, #10717, .T. ) ;
#20521=AXIS2_PLACEMENT_3D ( 'NONE', #8619, #220, #3334 ) ;
#20524=CYLINDRICAL_SURFACE ( 'NONE', #782, 0.5080000000000013394 ) ;
#20527=ORIENTED_EDGE ( 'NONE', *, *, #3462, .F. ) ;
#20534=AXIS2_PLACEMENT_3D ( 'NONE', #3848, #20398, #7040 ) ;
#20537=DIRECTION ( 'NONE',  ( 0.000000000000000000, 1.000000000000000000, -0.000000000000000000 ) ) ;
#20541=EDGE_CURVE ( 'NONE', #10543, #8326, #1353, .T. ) ;
#20545=CARTESIAN_POINT ( 'NONE',  ( 39.11079947626275555, -1.983739999999999837, -27.65534212225540500 ) ) ;
#20552=EDGE_LOOP ( 'NONE', ( #5573, #8482, #8261, #20519 ) ) ;
#20553=ORIENTED_EDGE ( 'NONE', *, *, #16504, .T. ) ;
#20561=CARTESIAN_POINT ( 'NONE',  ( 38.97455088732246509, 40.07865999999999929, -3.928096151774917999 ) ) ;
#20576=DIRECTION ( 'NONE',  ( 0.6496772031432432870, 0.000000000000000000, -0.7602101891687411683 ) ) ;
#20579=VECTOR ( 'NONE', #2405, 1000.000000000000114 ) ;
#20584=ORIENTED_EDGE ( 'NONE', *, *, #4268, .T. ) ;
#20586=CARTESIAN_POINT ( 'NONE',  ( 53.08681243024872742, 40.07829845791615497, -16.72443647849243575 ) ) ;
#20588=CARTESIAN_POINT ( 'NONE',  ( 52.49113927203449492, -6.356984999999999886, -16.14695822742181619 ) ) ;
#20589=VECTOR ( 'NONE', #8789, 1000.000000000000114 ) ;
#20594=ORIENTED_EDGE ( 'NONE', *, *, #2925, .F. ) ;
#20599=DIRECTION ( 'NONE',  ( 0.000000000000000000, -1.000000000000000000, -0.000000000000000000 ) ) ;
#20603=EDGE_LOOP ( 'NONE', ( #7688, #8501, #11353, #9631 ) ) ;
#20621=AXIS2_PLACEMENT_3D ( 'NONE', #1136, #14655, #21466 ) ;
#20623=CARTESIAN_POINT ( 'NONE',  ( 47.80475250345343596, -6.356985000000002550, -11.91473563638196786 ) ) ;
#20627=VERTEX_POINT ( 'NONE', #13082 ) ;
#20638=EDGE_LOOP ( 'NONE', ( #15375, #19090, #11797, #12239 ) ) ;
#20666=ORIENTED_EDGE ( 'NONE', *, *, #18457, .F. ) ;
#20667=ORIENTED_EDGE ( 'NONE', *, *, #21692, .F. ) ;
#20679=DIRECTION ( 'NONE',  ( 0.7421532822901579785, 0.000000000000000000, -0.6702301885068628895 ) ) ;
#20683=FACE_OUTER_BOUND ( 'NONE', #3490, .T. ) ;
#20688=DIRECTION ( 'NONE',  ( 0.000000000000000000, 1.000000000000000000, 0.000000000000000000 ) ) ;
#20692=EDGE_CURVE ( 'NONE', #3856, #14138, #10670, .T. ) ;
#20693=CARTESIAN_POINT ( 'NONE',  ( 61.56621290189396944, 29.95901653600000003, -0.7977859469341201937 ) ) ;
#20695=CARTESIAN_POINT ( 'NONE',  ( 42.35466991749225940, -9.531985000000000596, -17.94967221382040279 ) ) ;
#20697=EDGE_LOOP ( 'NONE', ( #6918, #19508, #13148, #13373 ) ) ;
#20699=EDGE_CURVE ( 'NONE', #1966, #1190, #19841, .T. ) ;
#20701=EDGE_CURVE ( 'NONE', #16977, #6777, #5191, .T. ) ;
#20705=ORIENTED_EDGE ( 'NONE', *, *, #3559, .F. ) ;
#20711=CARTESIAN_POINT ( 'NONE',  ( 30.50878709810603340, 32.54502000000000095, -19.83971405306587954 ) ) ;
#20714=EDGE_LOOP ( 'NONE', ( #651, #9139, #2528, #1556 ) ) ;
#20718=CARTESIAN_POINT ( 'NONE',  ( 41.78116128337411794, -4.569743463999999200, 7.392073290253172502 ) ) ;
#20721=CARTESIAN_POINT ( 'NONE',  ( 53.25483508941461963, 32.54501999999999384, -5.879799058943532941 ) ) ;
#20736=DIRECTION ( 'NONE',  ( 0.000000000000000000, -1.000000000000000000, -0.000000000000000000 ) ) ;
#20737=CARTESIAN_POINT ( 'NONE',  ( 53.84486179190094646, -76.79125307200000350, -6.412645463410259872 ) ) ;
#20746=EDGE_CURVE ( 'NONE', #17636, #10480, #18091, .T. ) ;
#20752=DIRECTION ( 'NONE',  ( 0.8667647648559581031, 0.000000000000000000, 0.4987171968201974948 ) ) ;
#20763=DIRECTION ( 'NONE',  ( 0.000000000000000000, -1.000000000000000000, -0.000000000000000000 ) ) ;
#20773=EDGE_LOOP ( 'NONE', ( #12426, #17918, #21009, #741 ) ) ;
#20775=DIRECTION ( 'NONE',  ( 0.4080888115384288528, 0.000000000000000000, 0.9129422336036122632 ) ) ;
#20777=ORIENTED_EDGE ( 'NONE', *, *, #19924, .F. ) ;
#20778=EDGE_LOOP ( 'NONE', ( #6048, #1690, #15030, #863 ) ) ;
#20780=CIRCLE ( 'NONE', #19012, 30.16249999999999076 ) ;
#20784=B_SPLINE_CURVE_WITH_KNOTS ( 'NONE', 3,
 ( #11471, #4837, #15127, #1508 ),
 .UNSPECIFIED., .F., .F.,
 ( 4, 4 ),
 ( 0.008535883516945940233, 0.009146310752443962550 ),
 .UNSPECIFIED. ) ;
#20794=LINE ( 'NONE', #4341, #6055 ) ;
#20798=AXIS2_PLACEMENT_3D ( 'NONE', #18625, #11896, #8251 ) ;
#20800=VERTEX_POINT ( 'NONE', #18571 ) ;
#20805=ORIENTED_EDGE ( 'NONE', *, *, #6584, .F. ) ;
#20808=CARTESIAN_POINT ( 'NONE',  ( 52.49113927203492125, -5.166360000000002728, -16.14695822742135078 ) ) ;
#20814=AXIS2_PLACEMENT_3D ( 'NONE', #13074, #18031, #19464 ) ;
#20819=CARTESIAN_POINT ( 'NONE',  ( 30.41963056417667488, -1.983739999999999837, -8.653862521447852174 ) ) ;
#20820=EDGE_CURVE ( 'NONE', #14694, #10716, #5292, .T. ) ;
#20825=CARTESIAN_POINT ( 'NONE',  ( 52.86938555161624009, 40.05505435406290360, -16.95752595126053919 ) ) ;
#20847=ORIENTED_EDGE ( 'NONE', *, *, #964, .F. ) ;
#20848=ADVANCED_FACE ( 'NONE', ( #14284 ), #2433, .T. ) ;
#20852=CARTESIAN_POINT ( 'NONE',  ( 44.27024749654656688, -9.531985000000000596, -8.722764363618033201 ) ) ;
#20857=AXIS2_PLACEMENT_3D ( 'NONE', #53, #13455, #7110 ) ;
#20864=ORIENTED_EDGE ( 'NONE', *, *, #8550, .T. ) ;
#20877=VERTEX_POINT ( 'NONE', #21002 ) ;
#20883=ORIENTED_EDGE ( 'NONE', *, *, #8174, .T. ) ;
#20887=FACE_OUTER_BOUND ( 'NONE', #12263, .T. ) ;
#20892=CARTESIAN_POINT ( 'NONE',  ( 38.28489021960990613, 38.88803500000000213, 2.732679409805250703 ) ) ;
#20893=CIRCLE ( 'NONE', #13853, 0.7950199999999993938 ) ;
#20894=AXIS2_PLACEMENT_3D ( 'NONE', #5075, #19884, #4756 ) ;
#20903=EDGE_CURVE ( 'NONE', #7959, #3770, #4330, .T. ) ;
#20908=CIRCLE ( 'NONE', #5373, 0.7950199999999993938 ) ;
#20909=DIRECTION ( 'NONE',  ( 0.6702301885068632226, 0.000000000000000000, 0.7421532822901576454 ) ) ;
#20913=CARTESIAN_POINT ( 'NONE',  ( 57.23009918853844624, 34.52875999999999834, -20.42665903041912401 ) ) ;
#20924=EDGE_LOOP ( 'NONE', ( #4863, #1095 ) ) ;
#20925=DIRECTION ( 'NONE',  ( -0.9959941601142525691, 0.000000000000000000, -0.08941830359777946935 ) ) ;
#20928=CARTESIAN_POINT ( 'NONE',  ( 49.28028498622276032, 32.54502000000000095, -25.68670502218146368 ) ) ;
#20933=VECTOR ( 'NONE', #9810, 1000.000000000000000 ) ;
#20946=AXIS2_PLACEMENT_3D ( 'NONE', #7598, #16233, #14585 ) ;
#20950=ORIENTED_EDGE ( 'NONE', *, *, #190, .F. ) ;
#20959=ORIENTED_EDGE ( 'NONE', *, *, #9073, .F. ) ;
#20964=AXIS2_PLACEMENT_3D ( 'NONE', #3425, #21669, #1546 ) ;
#20973=CYLINDRICAL_SURFACE ( 'NONE', #253, 9.524999999999998579 ) ;
#20978=ORIENTED_EDGE ( 'NONE', *, *, #5007, .T. ) ;
#20981=ORIENTED_EDGE ( 'NONE', *, *, #4449, .F. ) ;
#20989=EDGE_CURVE ( 'NONE', #20322, #11391, #15277, .T. ) ;
#20991=AXIS2_PLACEMENT_3D ( 'NONE', #5943, #12600, #10931 ) ;
#20992=B_SPLINE_CURVE_WITH_KNOTS ( 'NONE', 3,
 ( #9976, #21262, #11527, #11204, #18268, #9537, #4572, #11312, #348, #12079 ),
 .UNSPECIFIED., .F., .F.,
 ( 4, 2, 2, 2, 4 ),
 ( 0.0008058748238304858612, 0.001281964470574262520, 0.001758054117318039178, 0.002234143764061815619, 0.002710233410805592495 ),
 .UNSPECIFIED. ) ;
#20993=DIRECTION ( 'NONE',  ( 0.6702301885068632226, 0.000000000000000000, 0.7421532822901576454 ) ) ;
#21002=CARTESIAN_POINT ( 'NONE',  ( 53.25483508941461963, 0.000000000000000000, -5.879799058943532941 ) ) ;
#21006=CARTESIAN_POINT ( 'NONE',  ( 49.72033008250774344, 0.000000000000000000, -2.687827786179598277 ) ) ;
#21009=ORIENTED_EDGE ( 'NONE', *, *, #18748, .T. ) ;
#21016=DIRECTION ( 'NONE',  ( 0.000000000000000000, -1.000000000000000000, -0.000000000000000000 ) ) ;
#21021=AXIS2_PLACEMENT_3D ( 'NONE', #10991, #17747, #13928 ) ;
#21031=DIRECTION ( 'NONE',  ( 0.000000000000000000, 1.000000000000000000, 0.000000000000000000 ) ) ;
#21034=EDGE_CURVE ( 'NONE', #14160, #9035, #3625, .T. ) ;
#21035=DIRECTION ( 'NONE',  ( 0.000000000000000000, 1.000000000000000000, 0.000000000000000000 ) ) ;
#21036=EDGE_CURVE ( 'NONE', #2302, #18035, #20192, .T. ) ;
#21038=EDGE_CURVE ( 'NONE', #14138, #14787, #11262, .T. ) ;
#21041=ORIENTED_EDGE ( 'NONE', *, *, #10409, .F. ) ;
#21043=DIRECTION ( 'NONE',  ( 0.6702301885068630005, 0.000000000000000000, 0.7421532822901580895 ) ) ;
#21047=DIRECTION ( 'NONE',  ( 0.000000000000000000, -1.000000000000000000, -0.000000000000000000 ) ) ;
#21050=ORIENTED_EDGE ( 'NONE', *, *, #18858, .T. ) ;
#21053=ORIENTED_EDGE ( 'NONE', *, *, #3794, .T. ) ;
#21054=ADVANCED_FACE ( 'NONE', ( #9383 ), #881, .T. ) ;
#21062=DIRECTION ( 'NONE',  ( 0.000000000000000000, -1.000000000000000000, -0.000000000000000000 ) ) ;
#21063=CARTESIAN_POINT ( 'NONE',  ( 39.64154476330273269, -5.625436815413037195, -3.259749160125199108 ) ) ;
#21064=ORIENTED_EDGE ( 'NONE', *, *, #3055, .F. ) ;
#21068=CARTESIAN_POINT ( 'NONE',  ( 59.55063415577301811, -1.983739999999999837, -22.52230776719629191 ) ) ;
#21069=DIRECTION ( 'NONE',  ( 0.000000000000000000, -1.000000000000000000, -0.000000000000000000 ) ) ;
#21071=CARTESIAN_POINT ( 'NONE',  ( 61.83151161312219557, 0.000000000000000000, -0.3645647634491749334 ) ) ;
#21076=EDGE_LOOP ( 'NONE', ( #16855, #3661, #10328, #6170 ) ) ;
#21086=ORIENTED_EDGE ( 'NONE', *, *, #8951, .T. ) ;
#21091=CARTESIAN_POINT ( 'NONE',  ( 39.44501451162916084, 37.83287603509175767, -3.443458352271670631 ) ) ;
#21099=VERTEX_POINT ( 'NONE', #19075 ) ;
#21101=EDGE_CURVE ( 'NONE', #12400, #10833, #10329, .T. ) ;
#21118=EDGE_CURVE ( 'NONE', #13623, #9951, #13923, .T. ) ;
#21125=CARTESIAN_POINT ( 'NONE',  ( 53.10323493417986640, 40.07865999999999929, -16.70631907733998034 ) ) ;
#21126=DIRECTION ( 'NONE',  ( -0.6702301885068632226, 0.000000000000000000, -0.7421532822901576454 ) ) ;
#21130=CIRCLE ( 'NONE', #14451, 0.5079999999999984528 ) ;
#21131=EDGE_CURVE ( 'NONE', #7945, #2248, #5823, .T. ) ;
#21137=EDGE_LOOP ( 'NONE', ( #10442, #20883, #14942, #13200 ) ) ;
#21140=EDGE_CURVE ( 'NONE', #20877, #21393, #8911, .T. ) ;
#21141=DIRECTION ( 'NONE',  ( -0.07875956036501312318, 0.000000000000000000, 0.9968936410927243807 ) ) ;
#21142=CIRCLE ( 'NONE', #15172, 0.5080000000000001181 ) ;
#21146=EDGE_CURVE ( 'NONE', #21099, #18734, #5026, .T. ) ;
#21148=ADVANCED_FACE ( 'NONE', ( #15690 ), #7157, .T. ) ;
#21149=CARTESIAN_POINT ( 'NONE',  ( 42.27821610176829381, -1.983739999999999837, 7.496956594510385763 ) ) ;
#21151=CARTESIAN_POINT ( 'NONE',  ( 53.67193531911993176, -7.278946903169048355, -16.01476742963361843 ) ) ;
#21154=FACE_OUTER_BOUND ( 'NONE', #914, .T. ) ;
#21157=DIRECTION ( 'NONE',  ( -0.2227372614607790735, 0.000000000000000000, -0.9748785115884710528 ) ) ;
#21166=DIRECTION ( 'NONE',  ( 0.000000000000000000, 1.000000000000000000, 0.000000000000000000 ) ) ;
#21173=ORIENTED_EDGE ( 'NONE', *, *, #11498, .T. ) ;
#21175=LINE ( 'NONE', #6034, #12756 ) ;
#21176=EDGE_CURVE ( 'NONE', #2599, #17559, #1848, .T. ) ;
#21177=VECTOR ( 'NONE', #3691, 1000.000000000000114 ) ;
#21179=EDGE_LOOP ( 'NONE', ( #7239, #6497, #18869, #3415 ) ) ;
#21181=DIRECTION ( 'NONE',  ( -0.2064631973582987667, 0.000000000000000000, 0.9784543669157944601 ) ) ;
#21184=ORIENTED_EDGE ( 'NONE', *, *, #14121, .T. ) ;
#21190=ORIENTED_EDGE ( 'NONE', *, *, #13314, .T. ) ;
#21198=DIRECTION ( 'NONE',  ( 0.7421532822901572013, 0.000000000000000000, -0.6702301885068637777 ) ) ;
#21199=CARTESIAN_POINT ( 'NONE',  ( 39.59538228781720903, 37.96603874921844124, -3.302459560555300655 ) ) ;
#21205=VECTOR ( 'NONE', #19637, 1000.000000000000000 ) ;
#21206=PLANE ( 'NONE',  #11767 ) ;
#21209=DIRECTION ( 'NONE',  ( -0.8583349619704301325, 0.000000000000000000, 0.5130897514657842828 ) ) ;
#21211=VERTEX_POINT ( 'NONE', #2282 ) ;
#21216=VERTEX_POINT ( 'NONE', #9020 ) ;
#21217=ORIENTED_EDGE ( 'NONE', *, *, #5424, .T. ) ;
#21220=LINE ( 'NONE', #17822, #9099 ) ;
#21225=CARTESIAN_POINT ( 'NONE',  ( 59.90456643211351917, 32.54502000000000095, -2.926035437812116946 ) ) ;
#21226=ADVANCED_FACE ( 'NONE', ( #15796 ), #14251, .T. ) ;
#21227=AXIS2_PLACEMENT_3D ( 'NONE', #7198, #18895, #1983 ) ;
#21229=CIRCLE ( 'NONE', #1459, 30.16249999999998721 ) ;
#21230=CARTESIAN_POINT ( 'NONE',  ( 39.11079947626275555, 0.000000000000000000, -27.65534212225540500 ) ) ;
#21232=CYLINDRICAL_SURFACE ( 'NONE', #3529, 0.7950199999999985057 ) ;
#21237=DIRECTION ( 'NONE',  ( 0.000000000000000000, 1.000000000000000000, -0.000000000000000000 ) ) ;
#21240=CIRCLE ( 'NONE', #4302, 0.7950199999999988387 ) ;
#21252=CARTESIAN_POINT ( 'NONE',  ( 59.80894853325292360, -6.356984999999999886, -16.70545285374888778 ) ) ;
#21255=EDGE_CURVE ( 'NONE', #3908, #6597, #10690, .T. ) ;
#21257=AXIS2_PLACEMENT_3D ( 'NONE', #16988, #18636, #6928 ) ;
#21259=EDGE_CURVE ( 'NONE', #12951, #180, #10802, .T. ) ;
#21262=CARTESIAN_POINT ( 'NONE',  ( 38.18512253410862911, -6.196245922951924889, -4.927479914652647786 ) ) ;
#21271=VECTOR ( 'NONE', #16623, 1000.000000000000114 ) ;
#21278=FACE_OUTER_BOUND ( 'NONE', #3124, .T. ) ;
#21279=ORIENTED_EDGE ( 'NONE', *, *, #18927, .T. ) ;
#21284=ORIENTED_EDGE ( 'NONE', *, *, #3537, .T. ) ;
#21285=AXIS2_PLACEMENT_3D ( 'NONE', #18694, #10304, #8741 ) ;
#21287=ORIENTED_EDGE ( 'NONE', *, *, #2872, .F. ) ;
#21290=CYLINDRICAL_SURFACE ( 'NONE', #18601, 0.5080000000000000071 ) ;
#21293=ORIENTED_EDGE ( 'NONE', *, *, #7611, .T. ) ;
#21295=B_SPLINE_CURVE_WITH_KNOTS ( 'NONE', 3,
 ( #856, #7599, #20436, #15079 ),
 .UNSPECIFIED., .F., .F.,
 ( 4, 4 ),
 ( 0.008550247267032764359, 0.009162609743145760585 ),
 .UNSPECIFIED. ) ;
#21296=EDGE_LOOP ( 'NONE', ( #9361, #19340, #20132, #3720 ) ) ;
#21298=FACE_OUTER_BOUND ( 'NONE', #17351, .T. ) ;
#21304=VECTOR ( 'NONE', #10584, 1000.000000000000114 ) ;
#21314=CARTESIAN_POINT ( 'NONE',  ( 39.62791084302666178, -1.983739999999999837, -24.65774797299118859 ) ) ;
#21318=DIRECTION ( 'NONE',  ( 0.000000000000000000, 1.000000000000000000, 0.000000000000000000 ) ) ;
#21319=CARTESIAN_POINT ( 'NONE',  ( 49.41195815393805901, -9.531985000000000596, -1.411525001868561224 ) ) ;
#21320=CARTESIAN_POINT ( 'NONE',  ( 57.35354854712898742, 32.54502000000000095, -21.22263945788050776 ) ) ;
#21322=ORIENTED_EDGE ( 'NONE', *, *, #1772, .F. ) ;
#21331=EDGE_CURVE ( 'NONE', #1698, #2302, #15879, .T. ) ;
#21335=VECTOR ( 'NONE', #7347, 1000.000000000000114 ) ;
#21337=CYLINDRICAL_SURFACE ( 'NONE', #14991, 1.190624999999999822 ) ;
#21343=DIRECTION ( 'NONE',  ( 0.000000000000000000, 1.000000000000000000, 0.000000000000000000 ) ) ;
#21347=VERTEX_POINT ( 'NONE', #12322 ) ;
#21350=ORIENTED_EDGE ( 'NONE', *, *, #18827, .T. ) ;
#21363=CIRCLE ( 'NONE', #4777, 0.5079999999999997851 ) ;
#21368=DIRECTION ( 'NONE',  ( 0.000000000000000000, 1.000000000000000000, 0.000000000000000000 ) ) ;
#21375=DIRECTION ( 'NONE',  ( 0.000000000000000000, 1.000000000000000000, 0.000000000000000000 ) ) ;
#21376=LINE ( 'NONE', #12895, #1998 ) ;
#21387=DIRECTION ( 'NONE',  ( 0.000000000000000000, 1.000000000000000000, 0.000000000000000000 ) ) ;
#21389=ORIENTED_EDGE ( 'NONE', *, *, #8285, .T. ) ;
#21393=VERTEX_POINT ( 'NONE', #2259 ) ;
#21395=CARTESIAN_POINT ( 'NONE',  ( 38.57934937226391270, 39.92799049660965238, -4.392330771018444047 ) ) ;
#21399=SURFACE_STYLE_FILL_AREA ( #2956 ) ;
#21406=ADVANCED_FACE ( 'NONE', ( #5800 ), #7672, .T. ) ;
#21409=ORIENTED_EDGE ( 'NONE', *, *, #1701, .F. ) ;
#21422=EDGE_CURVE ( 'NONE', #10146, #19201, #3977, .T. ) ;
#21425=CARTESIAN_POINT ( 'NONE',  ( 38.60701496492545459, -1.983739999999999837, -26.94161103631838472 ) ) ;
#21426=FACE_OUTER_BOUND ( 'NONE', #20638, .T. ) ;
#21428=FACE_OUTER_BOUND ( 'NONE', #8082, .T. ) ;
#21429=EDGE_LOOP ( 'NONE', ( #11990, #948, #15056, #10894 ) ) ;
#21433=DIRECTION ( 'NONE',  ( 0.05085730733808393328, 0.000000000000000000, -0.9987059298363656357 ) ) ;
#21435=ORIENTED_EDGE ( 'NONE', *, *, #4379, .F. ) ;
#21450=CARTESIAN_POINT ( 'NONE',  ( 53.90573468513591138, -6.034543792452756072, -15.68687799581064013 ) ) ;
#21452=DIRECTION ( 'NONE',  ( 0.7532174416907910786, 0.000000000000000000, 0.6577716059034319773 ) ) ;
#21456=ORIENTED_EDGE ( 'NONE', *, *, #6683, .T. ) ;
#21461=DIRECTION ( 'NONE',  ( 0.4987171968201974948, 0.000000000000000000, -0.8667647648559582141 ) ) ;
#21466=DIRECTION ( 'NONE',  ( 0.000000000000000000, 1.000000000000000000, 0.000000000000000000 ) ) ;
#21475=CARTESIAN_POINT ( 'NONE',  ( 39.80203592816771874, 39.51271241376007737, -3.118117012970574198 ) ) ;
#21477=DIRECTION ( 'NONE',  ( -0.9943660382494290406, 0.000000000000000000, 0.1060008583745199739 ) ) ;
#21480=DIRECTION ( 'NONE',  ( 0.3542738219355897056, 0.000000000000000000, 0.9351417320872542627 ) ) ;
#21483=EDGE_CURVE ( 'NONE', #10146, #18443, #9432, .T. ) ;
#21486=CARTESIAN_POINT ( 'NONE',  ( 52.86882968722888876, 37.72141639867590612, -16.95806507629960791 ) ) ;
#21488=CARTESIAN_POINT ( 'NONE',  ( 47.80475250345343596, 42.06303499999999929, -11.91473563638196786 ) ) ;
#21489=VERTEX_POINT ( 'NONE', #1251 ) ;
#21491=B_SPLINE_CURVE_WITH_KNOTS ( 'NONE', 3,
 ( #6398, #13277, #16368, #20085, #1529, #13167, #19876, #3089, #1207, #16583, #4951, #7950, #4637, #1419, #14940, #18128, #14721, #11706 ),
 .UNSPECIFIED., .F., .F.,
 ( 4, 2, 2, 2, 2, 2, 2, 2, 4 ),
 ( 0.000000000000000000, 0.0004692937272967107249, 0.0009385874545934214499, 0.001407881181890132229, 0.001877174909186842900, 0.002346468636483553787, 0.002815762363780264458, 0.003285056091076975129, 0.003754349818373685799 ),
 .UNSPECIFIED. ) ;
#21492=CARTESIAN_POINT ( 'NONE',  ( 53.46798503507454825, -1.983739999999999837, 6.304111036318381878 ) ) ;
#21493=VECTOR ( 'NONE', #13596, 1000.000000000000114 ) ;
#21504=EDGE_CURVE ( 'NONE', #2030, #3173, #7991, .T. ) ;
#21506=CARTESIAN_POINT ( 'NONE',  ( 43.49132289107146931, -1.983739999999999837, 4.686923926377883021 ) ) ;
#21509=DIRECTION ( 'NONE',  ( -0.5222415575336509797, 0.000000000000000000, -0.8527976052879290281 ) ) ;
#21515=DIRECTION ( 'NONE',  ( -0.7421532822901579785, 0.000000000000000000, 0.6702301885068628895 ) ) ;
#21516=EDGE_LOOP ( 'NONE', ( #12155, #8704, #8934, #2419 ) ) ;
#21520=VERTEX_POINT ( 'NONE', #18063 ) ;
#21525=EDGE_CURVE ( 'NONE', #8118, #10568, #14432, .T. ) ;
#21528=MECHANICAL_DESIGN_GEOMETRIC_PRESENTATION_REPRESENTATION('',(#20112),#9877);
#21535=DIRECTION ( 'NONE',  ( 0.000000000000000000, 1.000000000000000000, 0.000000000000000000 ) ) ;
#21539=ORIENTED_EDGE ( 'NONE', *, *, #4646, .T. ) ;
#21547=VECTOR ( 'NONE', #15192, 1000.000000000000114 ) ;
#21551=EDGE_CURVE ( 'NONE', #19210, #7476, #13530, .T. ) ;
#21555=VECTOR ( 'NONE', #19990, 1000.000000000000114 ) ;
#21556=CIRCLE ( 'NONE', #4280, 9.524999999999996803 ) ;
#21557=CARTESIAN_POINT ( 'NONE',  ( 53.14266576735298031, -7.546379553159687781, -16.66242751532464084 ) ) ;
#21558=CYLINDRICAL_SURFACE ( 'NONE', #5982, 0.5080000000000001181 ) ;
#21574=DIRECTION ( 'NONE',  ( 0.000000000000000000, 1.000000000000000000, 0.000000000000000000 ) ) ;
#21585=CARTESIAN_POINT ( 'NONE',  ( 56.91751438644678984, 32.54502000000000095, -20.96198986413465448 ) ) ;
#21589=AXIS2_PLACEMENT_3D ( 'NONE', #10403, #17148, #19122 ) ;
#21591=CARTESIAN_POINT ( 'NONE',  ( 61.60152099976809126, 34.52875999999999834, -12.48877542598203405 ) ) ;
#21592=DIRECTION ( 'NONE',  ( -0.6702301885068639997, 0.000000000000000000, -0.7421532822901570903 ) ) ;
#21593=CARTESIAN_POINT ( 'NONE',  ( 64.14292646034530776, -1.983739999999999837, -12.24881465648521939 ) ) ;
#21594=CARTESIAN_POINT ( 'NONE',  ( 52.49113927203492125, -7.547609999999999708, -16.14695822742135078 ) ) ;
#21595=AXIS2_PLACEMENT_3D ( 'NONE', #4523, #16365, #12947 ) ;
#21596=EDGE_LOOP ( 'NONE', ( #4701, #4390, #16461, #7301 ) ) ;
#21597=LINE ( 'NONE', #18382, #9979 ) ;
#21598=DIRECTION ( 'NONE',  ( 0.000000000000000000, 1.000000000000000000, 0.000000000000000000 ) ) ;
#21599=VERTEX_POINT ( 'NONE', #11431 ) ;
#21605=FACE_OUTER_BOUND ( 'NONE', #8616, .T. ) ;
#21617=B_SPLINE_CURVE_WITH_KNOTS ( 'NONE', 3,
 ( #6687, #11781, #1175, #3380, #18400, #18093, #18204, #16762, #1278, #3056, #7915, #13132, #8019, #14689, #21395, #6249, #9780, #11664 ),
 .UNSPECIFIED., .F., .F.,
 ( 4, 2, 2, 2, 2, 2, 2, 2, 4 ),
 ( 0.003754349818373638095, 0.004223755935673031287, 0.004693162052972424045, 0.005162568170271817670, 0.005631974287571210429, 0.006101380404870604054, 0.006570786522169996813, 0.007040192639469389571, 0.007509598756768783197 ),
 .UNSPECIFIED. ) ;
#21631=VECTOR ( 'NONE', #12579, 1000.000000000000114 ) ;
#21633=DIRECTION ( 'NONE',  ( -0.000000000000000000, -1.000000000000000000, 0.000000000000000000 ) ) ;
#21639=VECTOR ( 'NONE', #10041, 1000.000000000000114 ) ;
#21659=LINE ( 'NONE', #16480, #4495 ) ;
#21660=EDGE_LOOP ( 'NONE', ( #2476, #1611, #1606, #5251 ) ) ;
#21669=DIRECTION ( 'NONE',  ( 0.000000000000000000, -1.000000000000000000, -0.000000000000000000 ) ) ;
#21674=ORIENTED_EDGE ( 'NONE', *, *, #10925, .F. ) ;
#21677=DIRECTION ( 'NONE',  ( -0.6702301885068628895, 0.000000000000000000, -0.7421532822901579785 ) ) ;
#21681=EDGE_LOOP ( 'NONE', ( #18131, #14965, #18535, #166, #7516 ) ) ;
#21687=AXIS2_PLACEMENT_3D ( 'NONE', #10778, #10671, #15880 ) ;
#21692=EDGE_CURVE ( 'NONE', #831, #2705, #12125, .T. ) ;
#21693=FACE_OUTER_BOUND ( 'NONE', #21516, .T. ) ;
#21704=CARTESIAN_POINT ( 'NONE',  ( 64.14292646034530776, 32.54502000000000095, -12.24881465648521939 ) ) ;
#21711=DIRECTION ( 'NONE',  ( 0.000000000000000000, -1.000000000000000000, -0.000000000000000000 ) ) ;
#21713=CARTESIAN_POINT ( 'NONE',  ( 42.66304184606194383, -9.531985000000000596, -19.22597499813143784 ) ) ;
#21721=VECTOR ( 'NONE', #18324, 1000.000000000000114 ) ;
#21722=CARTESIAN_POINT ( 'NONE',  ( 61.03378281434940078, 34.52875999999999834, -11.91737544536021431 ) ) ;
#21723=CARTESIAN_POINT ( 'NONE',  ( 27.93207353965470574, 34.52875999999999834, -8.388685343514779902 ) ) ;
#21734=FACE_OUTER_BOUND ( 'NONE', #10147, .T. ) ;
#21740=ORIENTED_EDGE ( 'NONE', *, *, #17069, .T. ) ;
#21747=FACE_BOUND ( 'NONE', #6046, .T. ) ;
#21751=DIRECTION ( 'NONE',  ( -0.6702301885068634446, 0.000000000000000000, -0.7421532822901576454 ) ) ;
#21756=DIRECTION ( 'NONE',  ( -0.5222415575336509797, 0.000000000000000000, -0.8527976052879290281 ) ) ;
#21760=EDGE_LOOP ( 'NONE', ( #8662, #17529, #14811, #11582 ) ) ;
#21766=DIRECTION ( 'NONE',  ( 0.4987171968201974948, 0.000000000000000000, -0.8667647648559581031 ) ) ;
#21768=ORIENTED_EDGE ( 'NONE', *, *, #16803, .F. ) ;
#21774=CARTESIAN_POINT ( 'NONE',  ( 39.27728671717661513, -1.983739999999999837, -23.95520057284206672 ) ) ;
#21776=ADVANCED_FACE ( 'NONE', ( #3241 ), #9978, .T. ) ;
#21778=AXIS2_PLACEMENT_3D ( 'NONE', #6458, #14553, #16428 ) ;
#21792=DIRECTION ( 'NONE',  ( 0.000000000000000000, -1.000000000000000000, -0.000000000000000000 ) ) ;
#21801=EDGE_CURVE ( 'NONE', #18960, #1819, #12476, .T. ) ;
#21818=CARTESIAN_POINT ( 'NONE',  ( 42.35466991749225940, -1.983739999999999837, -17.94967221382040279 ) ) ;
#21824=EDGE_CURVE ( 'NONE', #8918, #18428, #19355, .T. ) ;
#21837=EDGE_LOOP ( 'NONE', ( #2290, #15368, #20280, #4278 ) ) ;
#21842=EDGE_LOOP ( 'NONE', ( #6277, #12593, #13703, #19904 ) ) ;
#21843=VECTOR ( 'NONE', #4665, 1000.000000000000114 ) ;
#21852=CARTESIAN_POINT ( 'NONE',  ( 48.58367710892853353, 34.52875999999999834, -25.32442392637788231 ) ) ;
#21853=ORIENTED_EDGE ( 'NONE', *, *, #3741, .T. ) ;
#21860=AXIS2_PLACEMENT_3D ( 'NONE', #17667, #19635, #9248 ) ;
#21862=DIRECTION ( 'NONE',  ( -0.9987059298363656357, 0.000000000000000000, -0.05085730733808393328 ) ) ;
#21865=FACE_OUTER_BOUND ( 'NONE', #9283, .T. ) ;
#21872=EDGE_LOOP ( 'NONE', ( #9609, #3072, #17917, #15021 ) ) ;
#21873=ORIENTED_EDGE ( 'NONE', *, *, #4471, .F. ) ;
#21879=AXIS2_PLACEMENT_3D ( 'NONE', #8408, #20445, #15519 ) ;
ENDSEC;
END-ISO-10303-21;
